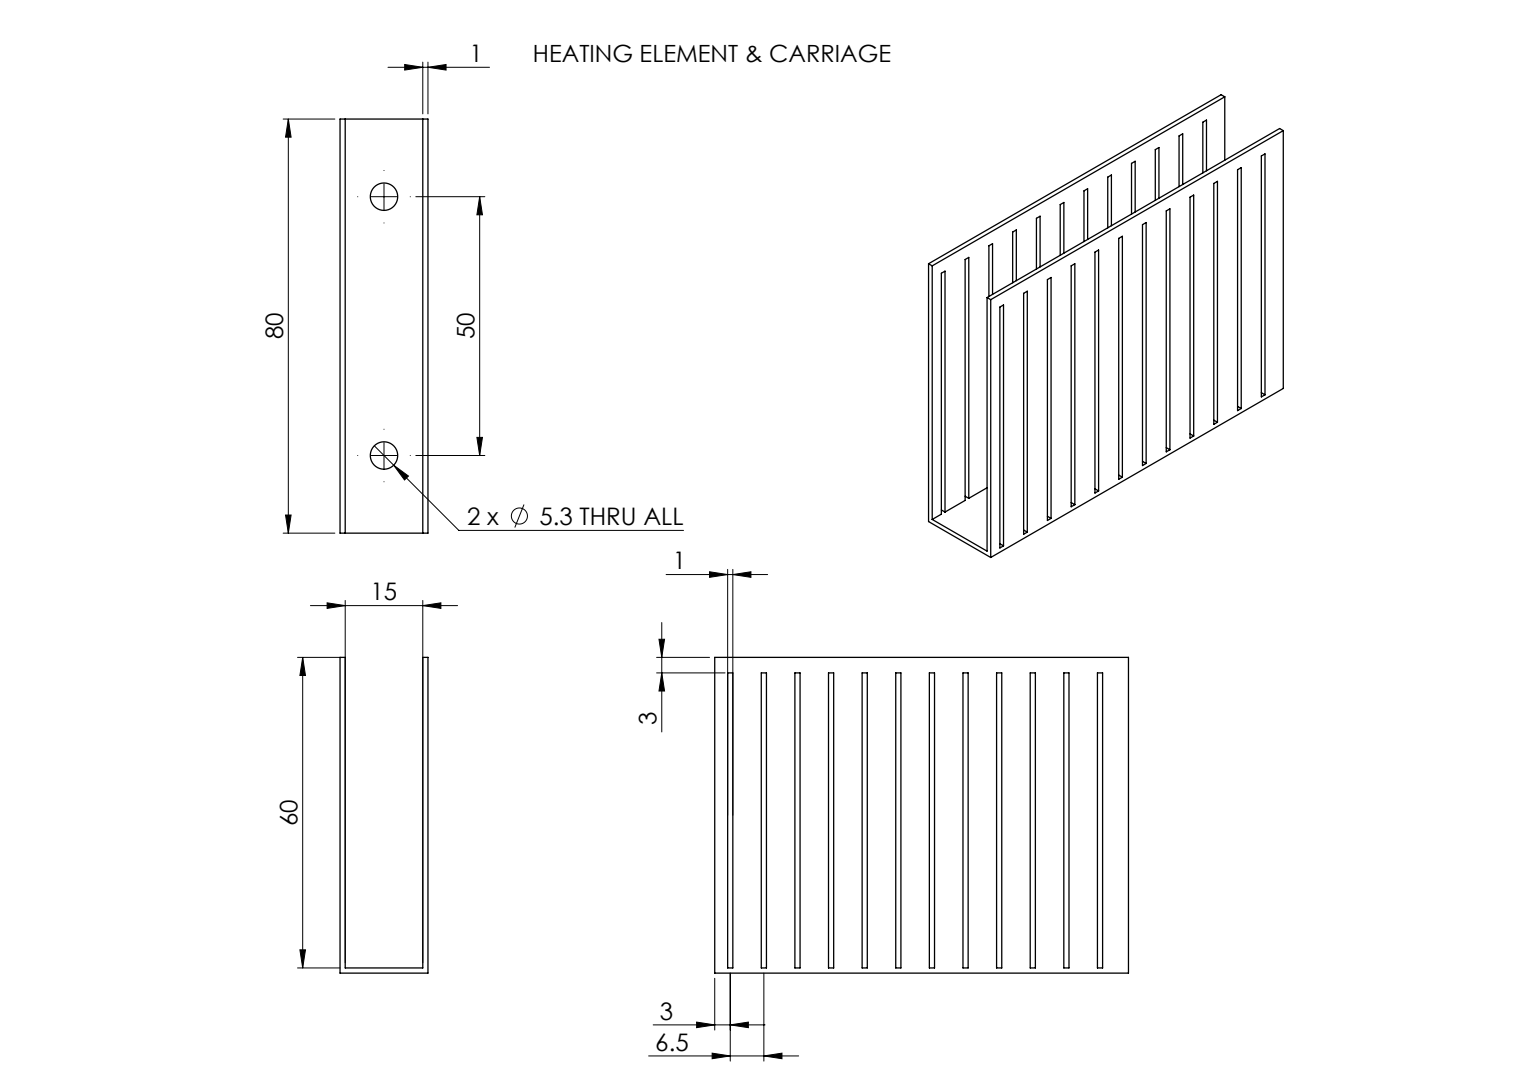
ISO-10303-21;
HEADER;
FILE_DESCRIPTION (('STEP AP214'),
    '1' );
FILE_NAME ('Heating Element & carriage.step',
    '2026-10-08T14:41:38',
    ( '' ),
    ( '' ),
    'SwSTEP 2.0',
    'SolidWorks 2026',
    '' );
FILE_SCHEMA (( 'AUTOMOTIVE_DESIGN' ));
ENDSEC;

DATA;
#2=VECTOR ( 'NONE', #8948, 1000.000000000000000 ) ;
#3=LINE ( 'NONE', #19320, #5933 ) ;
#8=DIRECTION ( 'NONE',  ( 0.000000000000000000, 0.000000000000000000, -1.000000000000000000 ) ) ;
#9=VERTEX_POINT ( 'NONE', #9196 ) ;
#11=VERTEX_POINT ( 'NONE', #7634 ) ;
#14=LINE ( 'NONE', #16487, #359 ) ;
#15=PRODUCT_CONTEXT ( 'NONE', #3327, 'mechanical' ) ;
#16=CARTESIAN_POINT ( 'NONE',  ( -25.00000000000000000, 53.00000000000000711, 30.00000000000000000 ) ) ;
#17=EDGE_CURVE ( 'NONE', #5613, #1380, #13300, .T. ) ;
#19=AXIS2_PLACEMENT_3D ( 'NONE', #7359, #17758, #4328 ) ;
#24=ORIENTED_EDGE ( 'NONE', *, *, #7353, .F. ) ;
#35=DIRECTION ( 'NONE',  ( -1.000000000000000000, 0.000000000000000000, -0.000000000000000000 ) ) ;
#39=CARTESIAN_POINT ( 'NONE',  ( -25.00000000000000000, 53.00000000000000711, -11.49999999999999645 ) ) ;
#46=PLANE ( 'NONE',  #8954 ) ;
#47=AXIS2_PLACEMENT_3D ( 'NONE', #8306, #16043, #2603 ) ;
#49=EDGE_LOOP ( 'NONE', ( #2329, #11638, #12440, #4824 ) ) ;
#60=CARTESIAN_POINT ( 'NONE',  ( -41.00000000000000711, 110.0000000000000000, 6.999999999999999112 ) ) ;
#64=EDGE_CURVE ( 'NONE', #9274, #14710, #15088, .T. ) ;
#67=AXIS2_PLACEMENT_3D ( 'NONE', #5864, #11526, #16244 ) ;
#76=VERTEX_POINT ( 'NONE', #16452 ) ;
#114=CARTESIAN_POINT ( 'NONE',  ( -24.00000000000000000, 53.00000000000000711, -18.00000000000000355 ) ) ;
#115=DIRECTION ( 'NONE',  ( 0.000000000000000000, 0.000000000000000000, -1.000000000000000000 ) ) ;
#130=ORIENTED_EDGE ( 'NONE', *, *, #2687, .F. ) ;
#132=EDGE_CURVE ( 'NONE', #16262, #13646, #5091, .T. ) ;
#141=DIRECTION ( 'NONE',  ( 0.000000000000000000, -1.000000000000000000, -0.000000000000000000 ) ) ;
#150=DIRECTION ( 'NONE',  ( 0.000000000000000000, 0.000000000000000000, 1.000000000000000000 ) ) ;
#173=ORIENTED_EDGE ( 'NONE', *, *, #18111, .T. ) ;
#176=CARTESIAN_POINT ( 'NONE',  ( -41.00000000000000711, 53.00000000000000711, 8.000000000000000000 ) ) ;
#184=VERTEX_POINT ( 'NONE', #3603 ) ;
#185=VERTEX_POINT ( 'NONE', #9574 ) ;
#193=VECTOR ( 'NONE', #5352, 1000.000000000000000 ) ;
#209=VERTEX_POINT ( 'NONE', #3697 ) ;
#218=CARTESIAN_POINT ( 'NONE',  ( -40.00000000000000000, 53.00000000000000711, 20.00000000000000000 ) ) ;
#221=LINE ( 'NONE', #319, #18355 ) ;
#230=EDGE_LOOP ( 'NONE', ( #8619, #14141, #10740, #17845 ) ) ;
#234=CARTESIAN_POINT ( 'NONE',  ( -40.00000000000000000, 53.00000000000000711, -32.00000000000000000 ) ) ;
#236=CARTESIAN_POINT ( 'NONE',  ( -41.00000000000000711, 53.00000000000000711, -45.00000000000000000 ) ) ;
#249=LINE ( 'NONE', #3293, #1715 ) ;
#254=CARTESIAN_POINT ( 'NONE',  ( -41.00000000000000711, 53.00000000000000711, 13.50000000000000000 ) ) ;
#258=EDGE_CURVE ( 'NONE', #10251, #6518, #1845, .T. ) ;
#277=ORIENTED_EDGE ( 'NONE', *, *, #8740, .F. ) ;
#279=CARTESIAN_POINT ( 'NONE',  ( -24.00000000000000711, 53.00000000000000711, -18.00000000000000000 ) ) ;
#280=EDGE_CURVE ( 'NONE', #3613, #17642, #1950, .T. ) ;
#285=EDGE_LOOP ( 'NONE', ( #7432, #10877, #13688, #10122 ) ) ;
#291=VERTEX_POINT ( 'NONE', #667 ) ;
#304=LINE ( 'NONE', #9218, #18172 ) ;
#309=LINE ( 'NONE', #12357, #13947 ) ;
#310=VECTOR ( 'NONE', #16083, 1000.000000000000000 ) ;
#313=VECTOR ( 'NONE', #8610, 1000.000000000000000 ) ;
#319=CARTESIAN_POINT ( 'NONE',  ( -40.00000000000000711, 110.0000000000000000, 30.00000000000000000 ) ) ;
#332=CARTESIAN_POINT ( 'NONE',  ( -25.00000000000000000, 113.0000000000000000, 30.00000000000000000 ) ) ;
#338=VECTOR ( 'NONE', #15976, 1000.000000000000000 ) ;
#342=AXIS2_PLACEMENT_3D ( 'NONE', #8168, #7978, #714 ) ;
#343=EDGE_LOOP ( 'NONE', ( #9305, #13118, #10006, #16658 ) ) ;
#349=FACE_OUTER_BOUND ( 'NONE', #18147, .T. ) ;
#353=DIRECTION ( 'NONE',  ( 1.000000000000000000, -0.000000000000000000, -0.000000000000000000 ) ) ;
#358=DIRECTION ( 'NONE',  ( 1.000000000000000000, -0.000000000000000000, -0.000000000000000000 ) ) ;
#359=VECTOR ( 'NONE', #18061, 1000.000000000000000 ) ;
#361=CARTESIAN_POINT ( 'NONE',  ( -41.00000000000000711, 53.00000000000000711, 27.50000000000000000 ) ) ;
#364=ORIENTED_EDGE ( 'NONE', *, *, #7937, .T. ) ;
#368=ORIENTED_EDGE ( 'NONE', *, *, #14861, .F. ) ;
#379=CARTESIAN_POINT ( 'NONE',  ( -25.00000000000000000, 53.00000000000000711, 30.00000000000000000 ) ) ;
#381=ORIENTED_EDGE ( 'NONE', *, *, #2414, .F. ) ;
#409=DIRECTION ( 'NONE',  ( 1.000000000000000000, -0.000000000000000000, -0.000000000000000000 ) ) ;
#412=CARTESIAN_POINT ( 'NONE',  ( -41.00000000000000711, 53.00000000000000711, 6.999999999999999112 ) ) ;
#417=DIRECTION ( 'NONE',  ( -0.000000000000000000, 1.000000000000000000, -0.000000000000000000 ) ) ;
#430=CARTESIAN_POINT ( 'NONE',  ( -41.00000000000000711, 110.0000000000000000, -6.000000000000001776 ) ) ;
#432=DIRECTION ( 'NONE',  ( 1.000000000000000000, -0.000000000000000000, -0.000000000000000000 ) ) ;
#436=EDGE_CURVE ( 'NONE', #19394, #6733, #8675, .T. ) ;
#437=CARTESIAN_POINT ( 'NONE',  ( -41.00000000000000711, 110.0000000000000000, 20.00000000000000000 ) ) ;
#453=ADVANCED_FACE ( 'NONE', ( #1229 ), #11327, .T. ) ;
#464=DIRECTION ( 'NONE',  ( 0.000000000000000000, -1.000000000000000000, 0.000000000000000000 ) ) ;
#472=VECTOR ( 'NONE', #8947, 1000.000000000000000 ) ;
#474=DIRECTION ( 'NONE',  ( 0.000000000000000000, 0.000000000000000000, 1.000000000000000000 ) ) ;
#478=LINE ( 'NONE', #15666, #7219 ) ;
#480=ORIENTED_EDGE ( 'NONE', *, *, #9077, .T. ) ;
#485=ORIENTED_EDGE ( 'NONE', *, *, #2062, .T. ) ;
#487=ORIENTED_EDGE ( 'NONE', *, *, #6763, .T. ) ;
#494=ORIENTED_EDGE ( 'NONE', *, *, #810, .F. ) ;
#499=CARTESIAN_POINT ( 'NONE',  ( -25.00000000000000711, 53.00000000000000711, 1.500000000000001332 ) ) ;
#501=FACE_BOUND ( 'NONE', #14667, .T. ) ;
#506=CARTESIAN_POINT ( 'NONE',  ( -41.00000000000000711, 53.00000000000000711, -45.00000000000000000 ) ) ;
#509=ORIENTED_EDGE ( 'NONE', *, *, #2274, .F. ) ;
#512=CARTESIAN_POINT ( 'NONE',  ( -41.00000000000000711, 53.00000000000000711, 26.50000000000000000 ) ) ;
#520=ORIENTED_EDGE ( 'NONE', *, *, #14321, .T. ) ;
#522=ORIENTED_EDGE ( 'NONE', *, *, #3988, .F. ) ;
#523=DIRECTION ( 'NONE',  ( -1.156482317317871478E-16, 1.000000000000000000, 0.000000000000000000 ) ) ;
#525=LINE ( 'NONE', #11565, #11597 ) ;
#529=VECTOR ( 'NONE', #12275, 1000.000000000000000 ) ;
#530=VECTOR ( 'NONE', #4637, 1000.000000000000000 ) ;
#532=DIRECTION ( 'NONE',  ( 0.000000000000000000, 0.000000000000000000, -1.000000000000000000 ) ) ;
#534=DIRECTION ( 'NONE',  ( 1.000000000000000000, -0.000000000000000000, -0.000000000000000000 ) ) ;
#564=LINE ( 'NONE', #18228, #7201 ) ;
#588=CARTESIAN_POINT ( 'NONE',  ( -41.00000000000000711, 53.00000000000000711, -24.49999999999999645 ) ) ;
#592=DIRECTION ( 'NONE',  ( -1.156482317317871478E-16, 1.000000000000000000, 0.000000000000000000 ) ) ;
#593=FACE_BOUND ( 'NONE', #7659, .T. ) ;
#599=VECTOR ( 'NONE', #2972, 1000.000000000000000 ) ;
#601=DIRECTION ( 'NONE',  ( 0.000000000000000000, 0.000000000000000000, -1.000000000000000000 ) ) ;
#605=ORIENTED_EDGE ( 'NONE', *, *, #6639, .T. ) ;
#612=VECTOR ( 'NONE', #474, 1000.000000000000000 ) ;
#617=ADVANCED_FACE ( 'NONE', ( #14763 ), #16425, .T. ) ;
#621=VECTOR ( 'NONE', #523, 1000.000000000000000 ) ;
#622=LINE ( 'NONE', #15618, #18616 ) ;
#625=EDGE_CURVE ( 'NONE', #3704, #982, #6141, .T. ) ;
#626=VECTOR ( 'NONE', #2257, 1000.000000000000000 ) ;
#630=AXIS2_PLACEMENT_3D ( 'NONE', #16972, #17154, #15490 ) ;
#634=VECTOR ( 'NONE', #11787, 1000.000000000000000 ) ;
#635=LINE ( 'NONE', #15629, #18156 ) ;
#643=CARTESIAN_POINT ( 'NONE',  ( -24.00000000000000000, 113.0000000000000000, 30.00000000000000000 ) ) ;
#645=VECTOR ( 'NONE', #16601, 1000.000000000000000 ) ;
#649=VECTOR ( 'NONE', #15920, 1000.000000000000000 ) ;
#650=ORIENTED_EDGE ( 'NONE', *, *, #9548, .F. ) ;
#656=EDGE_CURVE ( 'NONE', #10380, #10947, #3089, .T. ) ;
#658=FACE_OUTER_BOUND ( 'NONE', #6966, .T. ) ;
#659=EDGE_CURVE ( 'NONE', #16948, #10794, #10433, .T. ) ;
#664=EDGE_LOOP ( 'NONE', ( #7813, #9877, #10932, #13103 ) ) ;
#667=CARTESIAN_POINT ( 'NONE',  ( -41.00000000000000711, 110.0000000000000000, -32.00000000000000000 ) ) ;
#668=VECTOR ( 'NONE', #17005, 1000.000000000000000 ) ;
#670=CARTESIAN_POINT ( 'NONE',  ( -25.00000000000000000, 110.0000000000000000, 30.00000000000000000 ) ) ;
#678=ORIENTED_EDGE ( 'NONE', *, *, #14772, .F. ) ;
#681=ORIENTED_EDGE ( 'NONE', *, *, #18605, .T. ) ;
#689=ORIENTED_EDGE ( 'NONE', *, *, #866, .F. ) ;
#691=DIRECTION ( 'NONE',  ( 0.000000000000000000, -1.000000000000000000, -0.000000000000000000 ) ) ;
#692=ORIENTED_EDGE ( 'NONE', *, *, #7602, .T. ) ;
#695=CARTESIAN_POINT ( 'NONE',  ( -41.00000000000000711, 110.0000000000000000, -5.000000000000000888 ) ) ;
#707=ORIENTED_EDGE ( 'NONE', *, *, #2186, .T. ) ;
#710=ORIENTED_EDGE ( 'NONE', *, *, #11906, .T. ) ;
#714=DIRECTION ( 'NONE',  ( -1.000000000000000000, 0.000000000000000000, -0.000000000000000000 ) ) ;
#722=LINE ( 'NONE', #6702, #12252 ) ;
#726=ORIENTED_EDGE ( 'NONE', *, *, #2307, .T. ) ;
#733=CARTESIAN_POINT ( 'NONE',  ( -40.00000000000000000, 53.00000000000000711, 13.50000000000000000 ) ) ;
#735=DIRECTION ( 'NONE',  ( 0.000000000000000000, 0.000000000000000000, -1.000000000000000000 ) ) ;
#738=CARTESIAN_POINT ( 'NONE',  ( -41.00000000000000711, 53.00000000000000711, -19.00000000000000000 ) ) ;
#755=DIRECTION ( 'NONE',  ( 0.000000000000000000, 0.000000000000000000, -1.000000000000000000 ) ) ;
#758=VECTOR ( 'NONE', #9249, 1000.000000000000000 ) ;
#759=DIRECTION ( 'NONE',  ( 1.000000000000000000, -0.000000000000000000, -0.000000000000000000 ) ) ;
#760=EDGE_CURVE ( 'NONE', #2931, #1646, #7705, .T. ) ;
#766=ORIENTED_EDGE ( 'NONE', *, *, #2307, .F. ) ;
#767=ORIENTED_EDGE ( 'NONE', *, *, #16915, .F. ) ;
#773=LINE ( 'NONE', #2428, #11566 ) ;
#776=DIRECTION ( 'NONE',  ( 1.000000000000000000, -0.000000000000000000, -0.000000000000000000 ) ) ;
#778=DIRECTION ( 'NONE',  ( 0.000000000000000000, -1.000000000000000000, 0.000000000000000000 ) ) ;
#783=CARTESIAN_POINT ( 'NONE',  ( -40.00000000000000711, 113.0000000000000000, 6.999999999999999112 ) ) ;
#790=AXIS2_PLACEMENT_3D ( 'NONE', #8176, #5235, #14146 ) ;
#798=LINE ( 'NONE', #18747, #17206 ) ;
#802=VECTOR ( 'NONE', #3506, 1000.000000000000000 ) ;
#803=CARTESIAN_POINT ( 'NONE',  ( -41.00000000000000711, 110.0000000000000000, -5.000000000000000888 ) ) ;
#804=ORIENTED_EDGE ( 'NONE', *, *, #13435, .F. ) ;
#809=CARTESIAN_POINT ( 'NONE',  ( -41.00000000000000711, 113.0000000000000000, 30.00000000000000000 ) ) ;
#810=EDGE_CURVE ( 'NONE', #15519, #4628, #9647, .T. ) ;
#824=VECTOR ( 'NONE', #2637, 1000.000000000000000 ) ;
#836=VECTOR ( 'NONE', #15353, 1000.000000000000000 ) ;
#853=VERTEX_POINT ( 'NONE', #2582 ) ;
#857=ORIENTED_EDGE ( 'NONE', *, *, #3921, .T. ) ;
#864=CARTESIAN_POINT ( 'NONE',  ( -41.00000000000000711, 110.0000000000000000, 21.00000000000000000 ) ) ;
#866=EDGE_CURVE ( 'NONE', #19283, #17238, #6714, .T. ) ;
#868=PLANE ( 'NONE',  #16631 ) ;
#870=FACE_OUTER_BOUND ( 'NONE', #10505, .T. ) ;
#876=EDGE_CURVE ( 'NONE', #15646, #8090, #3962, .T. ) ;
#880=ORIENTED_EDGE ( 'NONE', *, *, #12234, .F. ) ;
#883=VECTOR ( 'NONE', #3984, 1000.000000000000000 ) ;
#890=EDGE_LOOP ( 'NONE', ( #5514, #15277, #16400, #16858 ) ) ;
#897=ADVANCED_FACE ( 'NONE', ( #8562 ), #18770, .T. ) ;
#901=SURFACE_STYLE_USAGE ( .BOTH. , #5326 ) ;
#906=EDGE_LOOP ( 'NONE', ( #5274, #17895, #7595, #10353 ) ) ;
#913=LINE ( 'NONE', #17382, #14105 ) ;
#916=LINE ( 'NONE', #1204, #4548 ) ;
#927=CARTESIAN_POINT ( 'NONE',  ( -41.00000000000000711, 110.0000000000000000, 14.50000000000000000 ) ) ;
#928=VECTOR ( 'NONE', #4321, 1000.000000000000000 ) ;
#934=PLANE ( 'NONE',  #16670 ) ;
#940=DIRECTION ( 'NONE',  ( 1.000000000000000000, 1.156482317317871478E-16, -0.000000000000000000 ) ) ;
#941=VECTOR ( 'NONE', #1797, 1000.000000000000000 ) ;
#943=LINE ( 'NONE', #17412, #883 ) ;
#944=FACE_OUTER_BOUND ( 'NONE', #1471, .T. ) ;
#950=ORIENTED_EDGE ( 'NONE', *, *, #18620, .F. ) ;
#952=FILL_AREA_STYLE_COLOUR ( '', #15246 ) ;
#967=AXIS2_PLACEMENT_3D ( 'NONE', #13487, #8976, #17705 ) ;
#968=FACE_OUTER_BOUND ( 'NONE', #890, .T. ) ;
#977=VECTOR ( 'NONE', #19393, 1000.000000000000000 ) ;
#978=CARTESIAN_POINT ( 'NONE',  ( -24.00000000000000711, 53.00000000000000711, 14.50000000000000000 ) ) ;
#981=EDGE_LOOP ( 'NONE', ( #1286, #11849, #18751, #17689 ) ) ;
#982=VERTEX_POINT ( 'NONE', #15919 ) ;
#993=VERTEX_POINT ( 'NONE', #12965 ) ;
#995=DIRECTION ( 'NONE',  ( -0.000000000000000000, -0.000000000000000000, -1.000000000000000000 ) ) ;
#998=DIRECTION ( 'NONE',  ( -1.156482317317871478E-16, 1.000000000000000000, 0.000000000000000000 ) ) ;
#1006=ADVANCED_FACE ( 'NONE', ( #4256 ), #4553, .F. ) ;
#1009=ORIENTED_EDGE ( 'NONE', *, *, #16981, .F. ) ;
#1017=DIRECTION ( 'NONE',  ( -0.000000000000000000, -0.000000000000000000, -1.000000000000000000 ) ) ;
#1029=LINE ( 'NONE', #3587, #8038 ) ;
#1034=PLANE ( 'NONE',  #12270 ) ;
#1042=LINE ( 'NONE', #15761, #17575 ) ;
#1049=VERTEX_POINT ( 'NONE', #13256 ) ;
#1050=VERTEX_POINT ( 'NONE', #3071 ) ;
#1054=CARTESIAN_POINT ( 'NONE',  ( -24.00000000000000000, 110.0000000000000000, 30.00000000000000000 ) ) ;
#1057=VERTEX_POINT ( 'NONE', #14943 ) ;
#1058=DIRECTION ( 'NONE',  ( 1.000000000000000000, -0.000000000000000000, -0.000000000000000000 ) ) ;
#1059=EDGE_LOOP ( 'NONE', ( #16999, #10652, #8275, #15172 ) ) ;
#1075=DIRECTION ( 'NONE',  ( 0.000000000000000000, 0.000000000000000000, 1.000000000000000000 ) ) ;
#1077=AXIS2_PLACEMENT_3D ( 'NONE', #3070, #4653, #6219 ) ;
#1094=CARTESIAN_POINT ( 'NONE',  ( -41.00000000000000711, 53.00000000000000711, 0.5000000000000004441 ) ) ;
#1096=PLANE ( 'NONE',  #13026 ) ;
#1106=EDGE_CURVE ( 'NONE', #3347, #18273, #16111, .T. ) ;
#1112=DIRECTION ( 'NONE',  ( -1.000000000000000000, 0.000000000000000000, -0.000000000000000000 ) ) ;
#1117=VECTOR ( 'NONE', #5853, 1000.000000000000000 ) ;
#1135=EDGE_CURVE ( 'NONE', #5597, #2911, #5918, .T. ) ;
#1141=VECTOR ( 'NONE', #9980, 1000.000000000000000 ) ;
#1143=DIRECTION ( 'NONE',  ( 1.000000000000000000, -0.000000000000000000, -0.000000000000000000 ) ) ;
#1161=LINE ( 'NONE', #15875, #6006 ) ;
#1167=DIRECTION ( 'NONE',  ( -0.000000000000000000, -0.000000000000000000, -1.000000000000000000 ) ) ;
#1173=ORIENTED_EDGE ( 'NONE', *, *, #3972, .F. ) ;
#1180=LINE ( 'NONE', #3749, #310 ) ;
#1184=CARTESIAN_POINT ( 'NONE',  ( -25.00000000000000000, 53.00000000000000711, -6.000000000000005329 ) ) ;
#1196=ADVANCED_FACE ( 'NONE', ( #5210 ), #3442, .T. ) ;
#1200=VERTEX_POINT ( 'NONE', #15692 ) ;
#1204=CARTESIAN_POINT ( 'NONE',  ( -24.00000000000000000, 53.00000000000000711, 30.00000000000000000 ) ) ;
#1212=DIRECTION ( 'NONE',  ( -1.156482317317871478E-16, 1.000000000000000000, 0.000000000000000000 ) ) ;
#1214=PLANE ( 'NONE',  #18980 ) ;
#1215=VECTOR ( 'NONE', #16726, 1000.000000000000000 ) ;
#1228=VECTOR ( 'NONE', #16896, 1000.000000000000000 ) ;
#1229=FACE_OUTER_BOUND ( 'NONE', #13960, .T. ) ;
#1233=DIRECTION ( 'NONE',  ( -1.000000000000000000, 0.000000000000000000, -0.000000000000000000 ) ) ;
#1236=VECTOR ( 'NONE', #8624, 1000.000000000000000 ) ;
#1241=EDGE_LOOP ( 'NONE', ( #11948, #10912, #17945, #1283, #1566, #9146, #520, #3733, #14803, #5855, #6245, #19227, #15301, #8219, #16469, #17525, #16503, #381, #18039, #7623, #19032, #7521, #5716, #16047, #880, #13494, #16643, #2727, #18760, #1009, #4004, #5780, #2228, #3499, #10444, #726, #9450, #8717, #10174, #15705, #13406, #9481, #5037, #3504, #6291, #11719, #4592, #1657, #18703, #12860, #1476, #9601, #14968, #5586, #12915, #1586, #15890, #10759, #2179, #173, #10361, #17542, #16573, #15103, #6064, #17514, #2445, #2873, #16154, #689, #364, #9395, #4625, #24, #10077, #11238, #16268, #11151, #19225, #9913, #15765, #10497, #6485, #19212, #5003, #15390, #7620, #10672, #10260, #6196, #7749, #1376, #485, #13117, #18781, #6011, #17055, #9084, #1773, #1677 ) ) ;
#1247=EDGE_LOOP ( 'NONE', ( #7632, #14235, #9399, #2813 ) ) ;
#1250=EDGE_CURVE ( 'NONE', #19005, #3857, #12736, .T. ) ;
#1253=AXIS2_PLACEMENT_3D ( 'NONE', #15002, #13527, #2941 ) ;
#1258=LINE ( 'NONE', #11829, #15370 ) ;
#1260=AXIS2_PLACEMENT_3D ( 'NONE', #5822, #17678, #1112 ) ;
#1273=VERTEX_POINT ( 'NONE', #15410 ) ;
#1274=EDGE_LOOP ( 'NONE', ( #8686, #17929, #678, #19092 ) ) ;
#1276=DIRECTION ( 'NONE',  ( 0.000000000000000000, 0.000000000000000000, -1.000000000000000000 ) ) ;
#1278=ORIENTED_EDGE ( 'NONE', *, *, #6601, .F. ) ;
#1281=VECTOR ( 'NONE', #16758, 1000.000000000000000 ) ;
#1282=CARTESIAN_POINT ( 'NONE',  ( -25.00000000000000000, 53.00000000000000711, 30.00000000000000000 ) ) ;
#1283=ORIENTED_EDGE ( 'NONE', *, *, #9412, .T. ) ;
#1286=ORIENTED_EDGE ( 'NONE', *, *, #9886, .T. ) ;
#1290=ORIENTED_EDGE ( 'NONE', *, *, #14321, .F. ) ;
#1291=CARTESIAN_POINT ( 'NONE',  ( -24.00000000000000711, 53.00000000000000711, 21.00000000000000000 ) ) ;
#1295=EDGE_CURVE ( 'NONE', #12537, #17031, #12824, .T. ) ;
#1310=VECTOR ( 'NONE', #18785, 1000.000000000000000 ) ;
#1312=ORIENTED_EDGE ( 'NONE', *, *, #15617, .F. ) ;
#1314=ORIENTED_EDGE ( 'NONE', *, *, #13054, .F. ) ;
#1317=DIRECTION ( 'NONE',  ( 0.000000000000000000, 0.000000000000000000, 1.000000000000000000 ) ) ;
#1335=DIRECTION ( 'NONE',  ( 0.000000000000000000, 0.000000000000000000, -1.000000000000000000 ) ) ;
#1337=DIRECTION ( 'NONE',  ( 1.000000000000000000, -0.000000000000000000, -0.000000000000000000 ) ) ;
#1342=ADVANCED_FACE ( 'NONE', ( #6586, #5295, #5122 ), #14307, .F. ) ;
#1343=CARTESIAN_POINT ( 'NONE',  ( -40.00000000000000711, 110.0000000000000000, 8.000000000000000000 ) ) ;
#1350=VERTEX_POINT ( 'NONE', #499 ) ;
#1352=CARTESIAN_POINT ( 'NONE',  ( -24.00000000000000000, 53.00000000000000711, 30.00000000000000000 ) ) ;
#1356=ORIENTED_EDGE ( 'NONE', *, *, #9299, .F. ) ;
#1368=CARTESIAN_POINT ( 'NONE',  ( -41.00000000000000711, 53.00000000000000711, 21.00000000000000000 ) ) ;
#1369=LINE ( 'NONE', #11947, #8007 ) ;
#1370=VERTEX_POINT ( 'NONE', #10978 ) ;
#1376=ORIENTED_EDGE ( 'NONE', *, *, #4289, .T. ) ;
#1380=VERTEX_POINT ( 'NONE', #9607 ) ;
#1384=EDGE_CURVE ( 'NONE', #7148, #3017, #15594, .T. ) ;
#1385=CARTESIAN_POINT ( 'NONE',  ( -25.00000000000000000, 113.0000000000000000, 30.00000000000000000 ) ) ;
#1386=ORIENTED_EDGE ( 'NONE', *, *, #13706, .F. ) ;
#1389=LINE ( 'NONE', #1492, #17894 ) ;
#1392=LINE ( 'NONE', #12066, #10527 ) ;
#1400=EDGE_CURVE ( 'NONE', #5597, #13388, #7241, .T. ) ;
#1408=FACE_OUTER_BOUND ( 'NONE', #2091, .T. ) ;
#1418=CARTESIAN_POINT ( 'NONE',  ( -25.00000000000000000, 53.00000000000000711, 1.500000000000001332 ) ) ;
#1421=ORIENTED_EDGE ( 'NONE', *, *, #15282, .F. ) ;
#1423=EDGE_CURVE ( 'NONE', #12114, #17652, #17346, .T. ) ;
#1425=DIRECTION ( 'NONE',  ( 0.000000000000000000, 0.000000000000000000, -1.000000000000000000 ) ) ;
#1439=FACE_OUTER_BOUND ( 'NONE', #11726, .T. ) ;
#1445=VECTOR ( 'NONE', #9654, 1000.000000000000000 ) ;
#1465=AXIS2_PLACEMENT_3D ( 'NONE', #512, #7971, #1987 ) ;
#1467=AXIS2_PLACEMENT_3D ( 'NONE', #4932, #18736, #5216 ) ;
#1468=LINE ( 'NONE', #18234, #16955 ) ;
#1471=EDGE_LOOP ( 'NONE', ( #15796, #4172, #5621, #13747 ) ) ;
#1475=CARTESIAN_POINT ( 'NONE',  ( -41.00000000000000711, 53.00000000000000711, -24.49999999999999645 ) ) ;
#1476=ORIENTED_EDGE ( 'NONE', *, *, #15747, .T. ) ;
#1479=EDGE_CURVE ( 'NONE', #4790, #1553, #4307, .T. ) ;
#1485=CARTESIAN_POINT ( 'NONE',  ( -24.00000000000000000, 52.00000000000000711, 30.00000000000000000 ) ) ;
#1492=CARTESIAN_POINT ( 'NONE',  ( -24.00000000000000000, 110.0000000000000000, 30.00000000000000000 ) ) ;
#1510=ORIENTED_EDGE ( 'NONE', *, *, #3396, .T. ) ;
#1518=EDGE_CURVE ( 'NONE', #3704, #12114, #13114, .T. ) ;
#1520=FACE_OUTER_BOUND ( 'NONE', #6704, .T. ) ;
#1532=DIRECTION ( 'NONE',  ( 1.000000000000000000, -0.000000000000000000, -0.000000000000000000 ) ) ;
#1534=CARTESIAN_POINT ( 'NONE',  ( -41.00000000000000711, 53.00000000000000711, 8.000000000000000000 ) ) ;
#1547=ORIENTED_EDGE ( 'NONE', *, *, #16219, .T. ) ;
#1553=VERTEX_POINT ( 'NONE', #5578 ) ;
#1566=ORIENTED_EDGE ( 'NONE', *, *, #11894, .F. ) ;
#1572=VERTEX_POINT ( 'NONE', #2625 ) ;
#1574=ORIENTED_EDGE ( 'NONE', *, *, #15403, .F. ) ;
#1577=AXIS2_PLACEMENT_3D ( 'NONE', #5121, #15303, #6392 ) ;
#1580=ORIENTED_EDGE ( 'NONE', *, *, #12249, .T. ) ;
#1582=EDGE_CURVE ( 'NONE', #16384, #14586, #19204, .T. ) ;
#1586=ORIENTED_EDGE ( 'NONE', *, *, #13525, .T. ) ;
#1589=LINE ( 'NONE', #114, #9423 ) ;
#1603=VECTOR ( 'NONE', #13229, 1000.000000000000000 ) ;
#1608=VECTOR ( 'NONE', #13834, 1000.000000000000000 ) ;
#1616=ADVANCED_FACE ( 'NONE', ( #10368 ), #17935, .T. ) ;
#1619=EDGE_CURVE ( 'NONE', #15030, #5693, #13303, .T. ) ;
#1620=AXIS2_PLACEMENT_3D ( 'NONE', #4076, #940, #8302 ) ;
#1623=AXIS2_PLACEMENT_3D ( 'NONE', #18592, #13139, #4034 ) ;
#1631=CARTESIAN_POINT ( 'NONE',  ( -24.00000000000000000, 53.00000000000000711, 30.00000000000000000 ) ) ;
#1634=EDGE_CURVE ( 'NONE', #19128, #291, #16456, .T. ) ;
#1639=LINE ( 'NONE', #12205, #13397 ) ;
#1646=VERTEX_POINT ( 'NONE', #279 ) ;
#1651=ORIENTED_EDGE ( 'NONE', *, *, #13062, .T. ) ;
#1653=LINE ( 'NONE', #1352, #15830 ) ;
#1657=ORIENTED_EDGE ( 'NONE', *, *, #14988, .T. ) ;
#1659=ORIENTED_EDGE ( 'NONE', *, *, #17, .T. ) ;
#1661=VERTEX_POINT ( 'NONE', #2925 ) ;
#1662=VERTEX_POINT ( 'NONE', #12233 ) ;
#1666=DIRECTION ( 'NONE',  ( 0.000000000000000000, 0.000000000000000000, -1.000000000000000000 ) ) ;
#1673=VERTEX_POINT ( 'NONE', #10756 ) ;
#1677=ORIENTED_EDGE ( 'NONE', *, *, #16225, .F. ) ;
#1685=CARTESIAN_POINT ( 'NONE',  ( -25.00000000000000000, 110.0000000000000000, 30.00000000000000000 ) ) ;
#1696=CARTESIAN_POINT ( 'NONE',  ( -41.00000000000000711, 53.00000000000000711, -32.00000000000000000 ) ) ;
#1705=VECTOR ( 'NONE', #14150, 1000.000000000000000 ) ;
#1715=VECTOR ( 'NONE', #6233, 1000.000000000000000 ) ;
#1725=DIRECTION ( 'NONE',  ( 0.000000000000000000, -1.000000000000000000, 0.000000000000000000 ) ) ;
#1727=DIRECTION ( 'NONE',  ( 0.000000000000000000, 0.000000000000000000, 1.000000000000000000 ) ) ;
#1728=EDGE_LOOP ( 'NONE', ( #18520, #15861, #6751, #2742 ) ) ;
#1734=DIRECTION ( 'NONE',  ( 1.000000000000000000, -0.000000000000000000, -0.000000000000000000 ) ) ;
#1735=ORIENTED_EDGE ( 'NONE', *, *, #7505, .F. ) ;
#1740=ORIENTED_EDGE ( 'NONE', *, *, #6968, .F. ) ;
#1751=DIRECTION ( 'NONE',  ( 0.000000000000000000, 0.000000000000000000, 1.000000000000000000 ) ) ;
#1752=DIRECTION ( 'NONE',  ( -0.000000000000000000, -0.000000000000000000, -1.000000000000000000 ) ) ;
#1756=CARTESIAN_POINT ( 'NONE',  ( -25.00000000000000000, 110.0000000000000000, 27.50000000000000000 ) ) ;
#1759=VECTOR ( 'NONE', #10320, 1000.000000000000000 ) ;
#1762=ORIENTED_EDGE ( 'NONE', *, *, #6968, .T. ) ;
#1767=VERTEX_POINT ( 'NONE', #9576 ) ;
#1768=ORIENTED_EDGE ( 'NONE', *, *, #5180, .F. ) ;
#1773=ORIENTED_EDGE ( 'NONE', *, *, #13926, .T. ) ;
#1780=ORIENTED_EDGE ( 'NONE', *, *, #14871, .T. ) ;
#1785=DIRECTION ( 'NONE',  ( 0.000000000000000000, -1.000000000000000000, -0.000000000000000000 ) ) ;
#1786=LINE ( 'NONE', #16, #13514 ) ;
#1791=AXIS2_PLACEMENT_3D ( 'NONE', #13713, #4815, #7646 ) ;
#1793=VERTEX_POINT ( 'NONE', #3414 ) ;
#1797=DIRECTION ( 'NONE',  ( 1.000000000000000000, -0.000000000000000000, -0.000000000000000000 ) ) ;
#1799=DIRECTION ( 'NONE',  ( 0.000000000000000000, 0.000000000000000000, -1.000000000000000000 ) ) ;
#1804=CARTESIAN_POINT ( 'NONE',  ( -41.00000000000000711, 53.00000000000000711, -6.000000000000001776 ) ) ;
#1805=CARTESIAN_POINT ( 'NONE',  ( -40.00000000000000000, 53.00000000000000711, 30.00000000000000000 ) ) ;
#1832=VERTEX_POINT ( 'NONE', #6368 ) ;
#1838=DIRECTION ( 'NONE',  ( 0.000000000000000000, 0.000000000000000000, -1.000000000000000000 ) ) ;
#1843=EDGE_LOOP ( 'NONE', ( #18532, #6957, #6275, #1278 ) ) ;
#1844=DIRECTION ( 'NONE',  ( 0.000000000000000000, 0.000000000000000000, -1.000000000000000000 ) ) ;
#1845=LINE ( 'NONE', #7831, #7893 ) ;
#1863=EDGE_LOOP ( 'NONE', ( #16180, #8342, #18695, #6665 ) ) ;
#1874=VERTEX_POINT ( 'NONE', #18525 ) ;
#1877=CARTESIAN_POINT ( 'NONE',  ( -40.00000000000000711, 53.00000000000000711, 8.000000000000000000 ) ) ;
#1878=EDGE_CURVE ( 'NONE', #1057, #15240, #18707, .T. ) ;
#1879=PLANE ( 'NONE',  #1577 ) ;
#1880=FACE_BOUND ( 'NONE', #1843, .T. ) ;
#1882=LINE ( 'NONE', #15501, #12863 ) ;
#1884=AXIS2_PLACEMENT_3D ( 'NONE', #13511, #17830, #3325 ) ;
#1890=ORIENTED_EDGE ( 'NONE', *, *, #760, .F. ) ;
#1893=ORIENTED_EDGE ( 'NONE', *, *, #12356, .T. ) ;
#1906=CARTESIAN_POINT ( 'NONE',  ( -41.00000000000000711, 53.00000000000000711, -44.00000000000000000 ) ) ;
#1908=AXIS2_PLACEMENT_3D ( 'NONE', #13111, #10073, #8704 ) ;
#1911=VECTOR ( 'NONE', #16871, 1000.000000000000000 ) ;
#1920=LINE ( 'NONE', #12489, #9763 ) ;
#1926=CARTESIAN_POINT ( 'NONE',  ( -25.00000000000000000, 53.00000000000000711, 30.00000000000000000 ) ) ;
#1929=DIRECTION ( 'NONE',  ( 0.000000000000000000, 0.000000000000000000, -1.000000000000000000 ) ) ;
#1931=AXIS2_PLACEMENT_3D ( 'NONE', #19330, #11859, #9026 ) ;
#1936=EDGE_LOOP ( 'NONE', ( #19049, #9020, #5575, #522 ) ) ;
#1939=ORIENTED_EDGE ( 'NONE', *, *, #18111, .F. ) ;
#1944=VECTOR ( 'NONE', #3202, 1000.000000000000000 ) ;
#1947=ORIENTED_EDGE ( 'NONE', *, *, #10082, .T. ) ;
#1950=LINE ( 'NONE', #8223, #12571 ) ;
#1958=EDGE_LOOP ( 'NONE', ( #17310, #17326, #17985, #14474 ) ) ;
#1987=DIRECTION ( 'NONE',  ( -1.000000000000000000, 0.000000000000000000, -0.000000000000000000 ) ) ;
#1992=FACE_OUTER_BOUND ( 'NONE', #7834, .T. ) ;
#1995=ORIENTED_EDGE ( 'NONE', *, *, #6514, .F. ) ;
#1996=LINE ( 'NONE', #7982, #621 ) ;
#2000=CARTESIAN_POINT ( 'NONE',  ( -41.00000000000000711, 53.00000000000000711, -45.00000000000000000 ) ) ;
#2008=( GEOMETRIC_REPRESENTATION_CONTEXT ( 3 ) GLOBAL_UNCERTAINTY_ASSIGNED_CONTEXT ( ( #3951 ) ) GLOBAL_UNIT_ASSIGNED_CONTEXT ( ( #4036, #14825, #15019 ) ) REPRESENTATION_CONTEXT ( 'NONE', 'WORKASPACE' ) );
#2009=CARTESIAN_POINT ( 'NONE',  ( -40.00000000000000000, 53.00000000000000711, -19.00000000000000000 ) ) ;
#2018=LINE ( 'NONE', #18305, #15413 ) ;
#2019=DIRECTION ( 'NONE',  ( -1.000000000000000000, 0.000000000000000000, -0.000000000000000000 ) ) ;
#2023=VECTOR ( 'NONE', #13859, 1000.000000000000000 ) ;
#2028=VERTEX_POINT ( 'NONE', #13078 ) ;
#2034=ORIENTED_EDGE ( 'NONE', *, *, #16815, .F. ) ;
#2038=DIRECTION ( 'NONE',  ( -1.156482317317871478E-16, 1.000000000000000000, 0.000000000000000000 ) ) ;
#2046=ORIENTED_EDGE ( 'NONE', *, *, #9532, .F. ) ;
#2049=CARTESIAN_POINT ( 'NONE',  ( -41.00000000000000711, 110.0000000000000000, 26.50000000000000000 ) ) ;
#2055=EDGE_CURVE ( 'NONE', #1767, #12537, #943, .T. ) ;
#2059=CARTESIAN_POINT ( 'NONE',  ( -24.00000000000000000, 110.0000000000000000, 19.99999999999999645 ) ) ;
#2062=EDGE_CURVE ( 'NONE', #17825, #12973, #3886, .T. ) ;
#2065=LINE ( 'NONE', #8056, #13773 ) ;
#2070=DIRECTION ( 'NONE',  ( 0.000000000000000000, 0.000000000000000000, -1.000000000000000000 ) ) ;
#2073=VECTOR ( 'NONE', #14569, 1000.000000000000000 ) ;
#2074=DIRECTION ( 'NONE',  ( 0.000000000000000000, 0.000000000000000000, -1.000000000000000000 ) ) ;
#2075=VECTOR ( 'NONE', #6244, 1000.000000000000000 ) ;
#2091=EDGE_LOOP ( 'NONE', ( #710, #277, #8234, #7127 ) ) ;
#2102=LINE ( 'NONE', #16904, #758 ) ;
#2106=ADVANCED_FACE ( 'NONE', ( #7115 ), #19078, .T. ) ;
#2112=DIRECTION ( 'NONE',  ( 0.000000000000000000, 0.000000000000000000, -1.000000000000000000 ) ) ;
#2120=CARTESIAN_POINT ( 'NONE',  ( -24.00000000000000000, 110.0000000000000000, 30.00000000000000000 ) ) ;
#2132=ORIENTED_EDGE ( 'NONE', *, *, #64, .T. ) ;
#2142=ORIENTED_EDGE ( 'NONE', *, *, #16219, .F. ) ;
#2146=VERTEX_POINT ( 'NONE', #17702 ) ;
#2150=VECTOR ( 'NONE', #11508, 1000.000000000000000 ) ;
#2153=CARTESIAN_POINT ( 'NONE',  ( -41.00000000000000711, 110.0000000000000000, -25.50000000000000000 ) ) ;
#2158=CARTESIAN_POINT ( 'NONE',  ( -41.00000000000000711, 53.00000000000000711, -6.000000000000001776 ) ) ;
#2162=CARTESIAN_POINT ( 'NONE',  ( -40.00000000000000000, 52.00000000000000711, 30.00000000000000000 ) ) ;
#2166=LINE ( 'NONE', #11258, #13473 ) ;
#2168=DIRECTION ( 'NONE',  ( 0.000000000000000000, 0.000000000000000000, 1.000000000000000000 ) ) ;
#2170=VERTEX_POINT ( 'NONE', #13675 ) ;
#2172=FACE_OUTER_BOUND ( 'NONE', #664, .T. ) ;
#2179=ORIENTED_EDGE ( 'NONE', *, *, #16558, .T. ) ;
#2181=CARTESIAN_POINT ( 'NONE',  ( -41.00000000000000711, 53.00000000000000711, 21.00000000000000000 ) ) ;
#2182=ORIENTED_EDGE ( 'NONE', *, *, #18397, .F. ) ;
#2184=FACE_OUTER_BOUND ( 'NONE', #3832, .T. ) ;
#2185=DIRECTION ( 'NONE',  ( 1.000000000000000000, -0.000000000000000000, -0.000000000000000000 ) ) ;
#2186=EDGE_CURVE ( 'NONE', #3115, #13282, #19372, .T. ) ;
#2203=EDGE_CURVE ( 'NONE', #1661, #2980, #5847, .T. ) ;
#2204=LINE ( 'NONE', #11019, #3903 ) ;
#2210=DIRECTION ( 'NONE',  ( 0.000000000000000000, -1.000000000000000000, 0.000000000000000000 ) ) ;
#2222=EDGE_CURVE ( 'NONE', #1572, #16704, #12004, .T. ) ;
#2228=ORIENTED_EDGE ( 'NONE', *, *, #12857, .F. ) ;
#2239=VERTEX_POINT ( 'NONE', #10630 ) ;
#2244=ORIENTED_EDGE ( 'NONE', *, *, #1518, .T. ) ;
#2245=ORIENTED_EDGE ( 'NONE', *, *, #8811, .F. ) ;
#2246=EDGE_CURVE ( 'NONE', #16262, #10297, #6239, .T. ) ;
#2252=DIRECTION ( 'NONE',  ( 0.000000000000000000, 0.000000000000000000, -1.000000000000000000 ) ) ;
#2257=DIRECTION ( 'NONE',  ( 0.000000000000000000, 0.000000000000000000, -1.000000000000000000 ) ) ;
#2266=VECTOR ( 'NONE', #15054, 1000.000000000000000 ) ;
#2269=VERTEX_POINT ( 'NONE', #2993 ) ;
#2274=EDGE_CURVE ( 'NONE', #9587, #17823, #1639, .T. ) ;
#2278=PLANE ( 'NONE',  #3150 ) ;
#2280=DIRECTION ( 'NONE',  ( -0.000000000000000000, -0.000000000000000000, -1.000000000000000000 ) ) ;
#2283=CARTESIAN_POINT ( 'NONE',  ( -40.00000000000000711, 113.0000000000000000, 1.500000000000001332 ) ) ;
#2285=FILL_AREA_STYLE ('',( #11474 ) ) ;
#2289=VERTEX_POINT ( 'NONE', #10435 ) ;
#2306=CARTESIAN_POINT ( 'NONE',  ( -41.00000000000000711, 110.0000000000000000, -12.50000000000000000 ) ) ;
#2307=EDGE_CURVE ( 'NONE', #14415, #6823, #17804, .T. ) ;
#2318=LINE ( 'NONE', #11505, #5595 ) ;
#2320=LINE ( 'NONE', #8304, #8422 ) ;
#2322=DIRECTION ( 'NONE',  ( -1.000000000000000000, 0.000000000000000000, -0.000000000000000000 ) ) ;
#2323=VECTOR ( 'NONE', #7393, 1000.000000000000000 ) ;
#2324=CARTESIAN_POINT ( 'NONE',  ( -25.00000000000000711, 53.00000000000000711, 0.5000000000000004441 ) ) ;
#2329=ORIENTED_EDGE ( 'NONE', *, *, #4305, .F. ) ;
#2340=CARTESIAN_POINT ( 'NONE',  ( -25.00000000000000000, 53.00000000000000711, -18.00000000000000355 ) ) ;
#2346=DIRECTION ( 'NONE',  ( 0.000000000000000000, 0.000000000000000000, -1.000000000000000000 ) ) ;
#2349=CARTESIAN_POINT ( 'NONE',  ( -41.00000000000000711, 110.0000000000000000, -5.000000000000000888 ) ) ;
#2354=LINE ( 'NONE', #10162, #338 ) ;
#2356=DIRECTION ( 'NONE',  ( 0.000000000000000000, 0.000000000000000000, -1.000000000000000000 ) ) ;
#2357=CARTESIAN_POINT ( 'NONE',  ( -24.00000000000000711, 53.00000000000000711, -30.99999999999999645 ) ) ;
#2358=VERTEX_POINT ( 'NONE', #11024 ) ;
#2381=VECTOR ( 'NONE', #19358, 1000.000000000000000 ) ;
#2398=EDGE_CURVE ( 'NONE', #18807, #19283, #18591, .T. ) ;
#2404=EDGE_CURVE ( 'NONE', #4659, #7333, #6343, .T. ) ;
#2407=EDGE_LOOP ( 'NONE', ( #11715, #12132, #2937, #4843 ) ) ;
#2414=EDGE_CURVE ( 'NONE', #15895, #11533, #15638, .T. ) ;
#2420=PRESENTATION_STYLE_ASSIGNMENT (( #5189 ) ) ;
#2423=ORIENTED_EDGE ( 'NONE', *, *, #14694, .F. ) ;
#2428=CARTESIAN_POINT ( 'NONE',  ( -41.00000000000000711, 53.00000000000000711, -38.50000000000000711 ) ) ;
#2439=EDGE_CURVE ( 'NONE', #7469, #17238, #5158, .T. ) ;
#2442=CARTESIAN_POINT ( 'NONE',  ( -41.00000000000000711, 110.0000000000000000, -30.99999999999999645 ) ) ;
#2444=ORIENTED_EDGE ( 'NONE', *, *, #7937, .F. ) ;
#2445=ORIENTED_EDGE ( 'NONE', *, *, #17190, .T. ) ;
#2448=DIRECTION ( 'NONE',  ( 0.000000000000000000, 0.000000000000000000, -1.000000000000000000 ) ) ;
#2449=ORIENTED_EDGE ( 'NONE', *, *, #5921, .T. ) ;
#2452=EDGE_CURVE ( 'NONE', #4121, #15591, #10734, .T. ) ;
#2456=CARTESIAN_POINT ( 'NONE',  ( -41.00000000000000711, 53.00000000000000711, -5.000000000000000888 ) ) ;
#2458=LINE ( 'NONE', #8631, #14071 ) ;
#2459=ORIENTED_EDGE ( 'NONE', *, *, #19083, .F. ) ;
#2460=CARTESIAN_POINT ( 'NONE',  ( -25.00000000000000000, 110.0000000000000000, 30.00000000000000000 ) ) ;
#2463=CARTESIAN_POINT ( 'NONE',  ( -41.00000000000000711, 53.00000000000000711, 20.00000000000000000 ) ) ;
#2465=DIRECTION ( 'NONE',  ( 0.000000000000000000, -1.000000000000000000, -0.000000000000000000 ) ) ;
#2486=VECTOR ( 'NONE', #13156, 1000.000000000000000 ) ;
#2488=CARTESIAN_POINT ( 'NONE',  ( -41.00000000000000711, 110.0000000000000000, 21.00000000000000000 ) ) ;
#2492=EDGE_CURVE ( 'NONE', #12636, #14875, #9834, .T. ) ;
#2497=LINE ( 'NONE', #8484, #1310 ) ;
#2512=CARTESIAN_POINT ( 'NONE',  ( -41.00000000000000711, 110.0000000000000000, 1.500000000000001332 ) ) ;
#2524=FACE_OUTER_BOUND ( 'NONE', #13829, .T. ) ;
#2527=ORIENTED_EDGE ( 'NONE', *, *, #2452, .T. ) ;
#2529=VECTOR ( 'NONE', #8495, 1000.000000000000000 ) ;
#2531=ORIENTED_EDGE ( 'NONE', *, *, #8652, .T. ) ;
#2540=FACE_OUTER_BOUND ( 'NONE', #8912, .T. ) ;
#2547=CARTESIAN_POINT ( 'NONE',  ( -41.00000000000000711, 53.00000000000000711, 26.50000000000000000 ) ) ;
#2566=DIRECTION ( 'NONE',  ( 1.000000000000000000, 1.156482317317871725E-16, -0.000000000000000000 ) ) ;
#2569=EDGE_CURVE ( 'NONE', #18998, #18134, #17590, .T. ) ;
#2574=EDGE_CURVE ( 'NONE', #4107, #4659, #7190, .T. ) ;
#2581=CARTESIAN_POINT ( 'NONE',  ( -41.00000000000000711, 53.00000000000000711, 26.50000000000000000 ) ) ;
#2582=CARTESIAN_POINT ( 'NONE',  ( -40.00000000000000711, 110.0000000000000000, -19.00000000000000355 ) ) ;
#2587=CARTESIAN_POINT ( 'NONE',  ( -32.50000000000000000, 53.00000000000000711, 15.00000000000000000 ) ) ;
#2590=VERTEX_POINT ( 'NONE', #4167 ) ;
#2603=DIRECTION ( 'NONE',  ( 0.000000000000000000, 0.000000000000000000, 1.000000000000000000 ) ) ;
#2605=CARTESIAN_POINT ( 'NONE',  ( -40.00000000000000711, 110.0000000000000000, 30.00000000000000000 ) ) ;
#2609=VERTEX_POINT ( 'NONE', #17007 ) ;
#2619=EDGE_LOOP ( 'NONE', ( #13810, #16935, #15387, #13295 ) ) ;
#2620=AXIS2_PLACEMENT_3D ( 'NONE', #809, #2566, #7074 ) ;
#2621=DIRECTION ( 'NONE',  ( -0.000000000000000000, -0.000000000000000000, -1.000000000000000000 ) ) ;
#2624=LINE ( 'NONE', #2349, #10921 ) ;
#2625=CARTESIAN_POINT ( 'NONE',  ( -41.00000000000000711, 53.00000000000000711, -30.99999999999999645 ) ) ;
#2632=EDGE_LOOP ( 'NONE', ( #9083, #4504, #1768, #9775 ) ) ;
#2637=DIRECTION ( 'NONE',  ( 0.000000000000000000, -1.000000000000000000, 0.000000000000000000 ) ) ;
#2638=ORIENTED_EDGE ( 'NONE', *, *, #16555, .F. ) ;
#2647=ORIENTED_EDGE ( 'NONE', *, *, #8995, .F. ) ;
#2649=ORIENTED_EDGE ( 'NONE', *, *, #17189, .T. ) ;
#2651=DIRECTION ( 'NONE',  ( -0.000000000000000000, -0.000000000000000000, -1.000000000000000000 ) ) ;
#2656=DIRECTION ( 'NONE',  ( -1.000000000000000000, 0.000000000000000000, -0.000000000000000000 ) ) ;
#2659=FACE_BOUND ( 'NONE', #11637, .T. ) ;
#2673=DIRECTION ( 'NONE',  ( 0.000000000000000000, 0.000000000000000000, -1.000000000000000000 ) ) ;
#2677=EDGE_CURVE ( 'NONE', #19215, #11338, #6321, .T. ) ;
#2685=PRODUCT_DEFINITION_SHAPE ( 'NONE', 'NONE',  #9182 ) ;
#2687=EDGE_CURVE ( 'NONE', #16539, #2590, #5044, .T. ) ;
#2698=EDGE_CURVE ( 'NONE', #15286, #14415, #16572, .T. ) ;
#2700=LINE ( 'NONE', #10432, #10637 ) ;
#2707=( GEOMETRIC_REPRESENTATION_CONTEXT ( 3 ) GLOBAL_UNCERTAINTY_ASSIGNED_CONTEXT ( ( #16714 ) ) GLOBAL_UNIT_ASSIGNED_CONTEXT ( ( #12339, #6186, #18241 ) ) REPRESENTATION_CONTEXT ( 'NONE', 'WORKASPACE' ) );
#2708=VECTOR ( 'NONE', #14350, 1000.000000000000000 ) ;
#2722=CARTESIAN_POINT ( 'NONE',  ( -32.50000000000000000, 53.00000000000000711, 17.64999999999998437 ) ) ;
#2727=ORIENTED_EDGE ( 'NONE', *, *, #7372, .T. ) ;
#2737=ORIENTED_EDGE ( 'NONE', *, *, #8879, .T. ) ;
#2742=ORIENTED_EDGE ( 'NONE', *, *, #16837, .F. ) ;
#2748=ORIENTED_EDGE ( 'NONE', *, *, #7353, .T. ) ;
#2754=PLANE ( 'NONE',  #12879 ) ;
#2782=VECTOR ( 'NONE', #4479, 1000.000000000000000 ) ;
#2797=VECTOR ( 'NONE', #5397, 1000.000000000000000 ) ;
#2798=CARTESIAN_POINT ( 'NONE',  ( -41.00000000000000711, 110.0000000000000000, 1.500000000000001332 ) ) ;
#2807=ORIENTED_EDGE ( 'NONE', *, *, #9847, .T. ) ;
#2810=EDGE_CURVE ( 'NONE', #16642, #6640, #12148, .T. ) ;
#2813=ORIENTED_EDGE ( 'NONE', *, *, #2492, .F. ) ;
#2832=EDGE_CURVE ( 'NONE', #1370, #6673, #7755, .T. ) ;
#2835=VERTEX_POINT ( 'NONE', #17850 ) ;
#2837=DIRECTION ( 'NONE',  ( 0.000000000000000000, 0.000000000000000000, -1.000000000000000000 ) ) ;
#2843=CARTESIAN_POINT ( 'NONE',  ( -24.00000000000000000, 53.00000000000000711, 21.00000000000000000 ) ) ;
#2844=ADVANCED_FACE ( 'NONE', ( #3041 ), #10679, .F. ) ;
#2854=FACE_OUTER_BOUND ( 'NONE', #12466, .T. ) ;
#2857=DIRECTION ( 'NONE',  ( -1.156482317317871478E-16, 1.000000000000000000, 0.000000000000000000 ) ) ;
#2863=ORIENTED_EDGE ( 'NONE', *, *, #8533, .T. ) ;
#2871=EDGE_LOOP ( 'NONE', ( #6456, #5564, #15323, #12070 ) ) ;
#2873=ORIENTED_EDGE ( 'NONE', *, *, #14905, .T. ) ;
#2876=LINE ( 'NONE', #2581, #2 ) ;
#2877=CARTESIAN_POINT ( 'NONE',  ( -41.00000000000000711, 110.0000000000000000, 20.00000000000000000 ) ) ;
#2881=FACE_BOUND ( 'NONE', #9818, .T. ) ;
#2886=EDGE_CURVE ( 'NONE', #13949, #5657, #9117, .T. ) ;
#2900=CARTESIAN_POINT ( 'NONE',  ( -40.00000000000000000, 53.00000000000000711, 30.00000000000000000 ) ) ;
#2906=PLANE ( 'NONE',  #10182 ) ;
#2907=ORIENTED_EDGE ( 'NONE', *, *, #12486, .F. ) ;
#2910=LINE ( 'NONE', #5956, #15679 ) ;
#2911=VERTEX_POINT ( 'NONE', #2059 ) ;
#2919=ORIENTED_EDGE ( 'NONE', *, *, #1250, .F. ) ;
#2925=CARTESIAN_POINT ( 'NONE',  ( -40.00000000000000000, 53.00000000000000711, 0.5000000000000004441 ) ) ;
#2931=VERTEX_POINT ( 'NONE', #7854 ) ;
#2937=ORIENTED_EDGE ( 'NONE', *, *, #659, .F. ) ;
#2941=DIRECTION ( 'NONE',  ( 0.000000000000000000, 0.000000000000000000, 1.000000000000000000 ) ) ;
#2944=CARTESIAN_POINT ( 'NONE',  ( -40.00000000000000711, 113.0000000000000000, -45.00000000000000000 ) ) ;
#2955=MECHANICAL_DESIGN_GEOMETRIC_PRESENTATION_REPRESENTATION('',(#14850),#2008);
#2956=CARTESIAN_POINT ( 'NONE',  ( -41.00000000000000711, 53.00000000000000711, 14.50000000000000000 ) ) ;
#2959=ORIENTED_EDGE ( 'NONE', *, *, #11929, .F. ) ;
#2972=DIRECTION ( 'NONE',  ( 0.000000000000000000, -1.000000000000000000, 0.000000000000000000 ) ) ;
#2980=VERTEX_POINT ( 'NONE', #3716 ) ;
#2991=VECTOR ( 'NONE', #11645, 1000.000000000000000 ) ;
#2993=CARTESIAN_POINT ( 'NONE',  ( -25.00000000000000711, 110.0000000000000000, 6.999999999999999112 ) ) ;
#2994=EDGE_CURVE ( 'NONE', #12352, #18999, #18441, .T. ) ;
#3017=VERTEX_POINT ( 'NONE', #5009 ) ;
#3018=LINE ( 'NONE', #13299, #18825 ) ;
#3022=DIRECTION ( 'NONE',  ( 0.000000000000000000, 1.000000000000000000, 0.000000000000000000 ) ) ;
#3023=ADVANCED_FACE ( 'NONE', ( #12254 ), #10968, .T. ) ;
#3027=CARTESIAN_POINT ( 'NONE',  ( -40.00000000000000711, 110.0000000000000000, 30.00000000000000000 ) ) ;
#3039=ADVANCED_FACE ( 'NONE', ( #9501 ), #11064, .T. ) ;
#3041=FACE_OUTER_BOUND ( 'NONE', #4414, .T. ) ;
#3042=EDGE_LOOP ( 'NONE', ( #2907, #7887, #6384, #15431 ) ) ;
#3048=ORIENTED_EDGE ( 'NONE', *, *, #16453, .F. ) ;
#3053=DIRECTION ( 'NONE',  ( -1.156482317317871478E-16, 1.000000000000000000, 0.000000000000000000 ) ) ;
#3055=DIRECTION ( 'NONE',  ( 0.000000000000000000, -1.000000000000000000, 0.000000000000000000 ) ) ;
#3070=CARTESIAN_POINT ( 'NONE',  ( -41.00000000000000711, 53.00000000000000711, -30.99999999999999645 ) ) ;
#3071=CARTESIAN_POINT ( 'NONE',  ( -25.00000000000000000, 113.0000000000000000, -50.00000000000000000 ) ) ;
#3089=LINE ( 'NONE', #17907, #18761 ) ;
#3096=LINE ( 'NONE', #927, #18665 ) ;
#3097=EDGE_CURVE ( 'NONE', #6553, #9106, #773, .T. ) ;
#3098=CARTESIAN_POINT ( 'NONE',  ( -40.00000000000000711, 110.0000000000000000, 14.50000000000000000 ) ) ;
#3101=EDGE_LOOP ( 'NONE', ( #19144, #17751, #13426, #18140 ) ) ;
#3103=VECTOR ( 'NONE', #8262, 1000.000000000000000 ) ;
#3106=EDGE_LOOP ( 'NONE', ( #14869, #7316, #14335, #3048 ) ) ;
#3107=ORIENTED_EDGE ( 'NONE', *, *, #16225, .T. ) ;
#3115=VERTEX_POINT ( 'NONE', #4102 ) ;
#3116=ORIENTED_EDGE ( 'NONE', *, *, #7505, .T. ) ;
#3117=LINE ( 'NONE', #7330, #977 ) ;
#3127=EDGE_LOOP ( 'NONE', ( #7341, #13695, #17840, #4878 ) ) ;
#3133=VECTOR ( 'NONE', #11633, 1000.000000000000000 ) ;
#3136=EDGE_CURVE ( 'NONE', #6673, #15600, #5474, .T. ) ;
#3139=CARTESIAN_POINT ( 'NONE',  ( -41.00000000000000711, 53.00000000000000711, -12.50000000000000000 ) ) ;
#3140=ORIENTED_EDGE ( 'NONE', *, *, #11983, .F. ) ;
#3148=DIRECTION ( 'NONE',  ( 0.000000000000000000, 0.000000000000000000, -1.000000000000000000 ) ) ;
#3150=AXIS2_PLACEMENT_3D ( 'NONE', #8537, #6969, #14324 ) ;
#3151=LINE ( 'NONE', #9515, #8966 ) ;
#3152=DIRECTION ( 'NONE',  ( 0.000000000000000000, -1.000000000000000000, 0.000000000000000000 ) ) ;
#3157=EDGE_CURVE ( 'NONE', #2911, #15600, #13100, .T. ) ;
#3167=DIRECTION ( 'NONE',  ( 0.000000000000000000, 0.000000000000000000, -1.000000000000000000 ) ) ;
#3171=VERTEX_POINT ( 'NONE', #2722 ) ;
#3173=LINE ( 'NONE', #11785, #472 ) ;
#3174=VECTOR ( 'NONE', #4385, 1000.000000000000000 ) ;
#3175=CARTESIAN_POINT ( 'NONE',  ( -24.00000000000000711, 53.00000000000000711, -44.00000000000000000 ) ) ;
#3178=ADVANCED_FACE ( 'NONE', ( #15776 ), #17337, .T. ) ;
#3179=CARTESIAN_POINT ( 'NONE',  ( -24.00000000000000000, 53.00000000000000711, -44.00000000000000000 ) ) ;
#3185=AXIS2_PLACEMENT_3D ( 'NONE', #8363, #2465, #5510 ) ;
#3195=DIRECTION ( 'NONE',  ( -0.000000000000000000, 1.000000000000000000, -0.000000000000000000 ) ) ;
#3201=VECTOR ( 'NONE', #9235, 1000.000000000000000 ) ;
#3202=DIRECTION ( 'NONE',  ( 1.000000000000000000, -0.000000000000000000, -0.000000000000000000 ) ) ;
#3205=CARTESIAN_POINT ( 'NONE',  ( -41.00000000000000711, 53.00000000000000711, -45.00000000000000000 ) ) ;
#3223=EDGE_LOOP ( 'NONE', ( #5305, #12286, #13981, #2245 ) ) ;
#3231=ORIENTED_EDGE ( 'NONE', *, *, #16480, .F. ) ;
#3235=ORIENTED_EDGE ( 'NONE', *, *, #4338, .F. ) ;
#3240=CARTESIAN_POINT ( 'NONE',  ( -41.00000000000000711, 53.00000000000000711, 6.999999999999999112 ) ) ;
#3252=PLANE ( 'NONE',  #8645 ) ;
#3254=ADVANCED_FACE ( 'NONE', ( #19004 ), #6757, .T. ) ;
#3261=LINE ( 'NONE', #9232, #17730 ) ;
#3264=EDGE_CURVE ( 'NONE', #16948, #4790, #17040, .T. ) ;
#3293=CARTESIAN_POINT ( 'NONE',  ( -24.00000000000000000, 110.0000000000000000, 30.00000000000000000 ) ) ;
#3296=LINE ( 'NONE', #4672, #9754 ) ;
#3301=VECTOR ( 'NONE', #12288, 1000.000000000000000 ) ;
#3306=EDGE_LOOP ( 'NONE', ( #5461, #1780, #9762, #9494 ) ) ;
#3315=VECTOR ( 'NONE', #19336, 1000.000000000000000 ) ;
#3316=AXIS2_PLACEMENT_3D ( 'NONE', #5169, #8214, #5082 ) ;
#3325=DIRECTION ( 'NONE',  ( -1.000000000000000000, 0.000000000000000000, -0.000000000000000000 ) ) ;
#3326=LINE ( 'NONE', #13701, #4435 ) ;
#3327=APPLICATION_CONTEXT ( 'automotive_design' ) ;
#3328=DIRECTION ( 'NONE',  ( 0.000000000000000000, -1.000000000000000000, 0.000000000000000000 ) ) ;
#3334=ORIENTED_EDGE ( 'NONE', *, *, #5808, .T. ) ;
#3342=CARTESIAN_POINT ( 'NONE',  ( -41.00000000000000711, 110.0000000000000000, -24.49999999999999645 ) ) ;
#3347=VERTEX_POINT ( 'NONE', #12869 ) ;
#3354=LINE ( 'NONE', #13927, #4875 ) ;
#3357=DIRECTION ( 'NONE',  ( 0.000000000000000000, 1.000000000000000000, 0.000000000000000000 ) ) ;
#3363=LINE ( 'NONE', #3645, #529 ) ;
#3367=ORIENTED_EDGE ( 'NONE', *, *, #4746, .T. ) ;
#3368=DIRECTION ( 'NONE',  ( -1.000000000000000000, 0.000000000000000000, -0.000000000000000000 ) ) ;
#3372=CARTESIAN_POINT ( 'NONE',  ( -41.00000000000000711, 110.0000000000000000, -5.000000000000004441 ) ) ;
#3381=EDGE_CURVE ( 'NONE', #18025, #17238, #913, .T. ) ;
#3385=DIRECTION ( 'NONE',  ( -1.000000000000000000, 0.000000000000000000, -0.000000000000000000 ) ) ;
#3390=DIRECTION ( 'NONE',  ( 1.000000000000000000, -0.000000000000000000, -0.000000000000000000 ) ) ;
#3391=LINE ( 'NONE', #9362, #836 ) ;
#3395=EDGE_CURVE ( 'NONE', #9366, #7944, #9917, .T. ) ;
#3396=EDGE_CURVE ( 'NONE', #7331, #4488, #6019, .T. ) ;
#3399=ADVANCED_FACE ( 'NONE', ( #16399 ), #5816, .F. ) ;
#3404=CARTESIAN_POINT ( 'NONE',  ( -41.00000000000000711, 110.0000000000000000, -12.50000000000000000 ) ) ;
#3410=AXIS2_PLACEMENT_3D ( 'NONE', #4278, #11806, #1335 ) ;
#3414=CARTESIAN_POINT ( 'NONE',  ( -40.00000000000000711, 53.00000000000000711, 21.00000000000000000 ) ) ;
#3416=CARTESIAN_POINT ( 'NONE',  ( -25.00000000000000000, 53.00000000000000711, -12.49999999999999645 ) ) ;
#3436=ORIENTED_EDGE ( 'NONE', *, *, #1878, .T. ) ;
#3442=PLANE ( 'NONE',  #6856 ) ;
#3445=CARTESIAN_POINT ( 'NONE',  ( -25.00000000000000711, 53.00000000000000711, 8.000000000000000000 ) ) ;
#3449=DIRECTION ( 'NONE',  ( -1.156482317317871478E-16, 1.000000000000000000, 0.000000000000000000 ) ) ;
#3458=EDGE_CURVE ( 'NONE', #10251, #10640, #17772, .T. ) ;
#3461=LINE ( 'NONE', #18569, #941 ) ;
#3464=LINE ( 'NONE', #12378, #9375 ) ;
#3465=ORIENTED_EDGE ( 'NONE', *, *, #7972, .F. ) ;
#3470=EDGE_CURVE ( 'NONE', #982, #17652, #9398, .T. ) ;
#3484=DIRECTION ( 'NONE',  ( -1.156482317317871478E-16, 1.000000000000000000, 0.000000000000000000 ) ) ;
#3489=DIRECTION ( 'NONE',  ( 0.000000000000000000, 0.000000000000000000, -1.000000000000000000 ) ) ;
#3492=LINE ( 'NONE', #9466, #2708 ) ;
#3494=EDGE_CURVE ( 'NONE', #2269, #15646, #4648, .T. ) ;
#3499=ORIENTED_EDGE ( 'NONE', *, *, #13062, .F. ) ;
#3504=ORIENTED_EDGE ( 'NONE', *, *, #9649, .T. ) ;
#3506=DIRECTION ( 'NONE',  ( 1.000000000000000000, -0.000000000000000000, -0.000000000000000000 ) ) ;
#3509=VECTOR ( 'NONE', #3053, 1000.000000000000000 ) ;
#3528=VERTEX_POINT ( 'NONE', #7474 ) ;
#3533=ORIENTED_EDGE ( 'NONE', *, *, #656, .T. ) ;
#3548=DIRECTION ( 'NONE',  ( -0.000000000000000000, 1.000000000000000000, -0.000000000000000000 ) ) ;
#3549=DIRECTION ( 'NONE',  ( 0.000000000000000000, -1.000000000000000000, 0.000000000000000000 ) ) ;
#3553=LINE ( 'NONE', #7774, #7402 ) ;
#3559=CARTESIAN_POINT ( 'NONE',  ( -41.00000000000000711, 110.0000000000000000, 27.50000000000000000 ) ) ;
#3562=DIRECTION ( 'NONE',  ( 0.000000000000000000, 0.000000000000000000, 1.000000000000000000 ) ) ;
#3571=EDGE_CURVE ( 'NONE', #4981, #12140, #3461, .T. ) ;
#3574=COLOUR_RGB ( '', 0.72549020, 0.75294118, 0.79215686) ;
#3575=DIRECTION ( 'NONE',  ( 0.000000000000000000, 0.000000000000000000, -1.000000000000000000 ) ) ;
#3587=CARTESIAN_POINT ( 'NONE',  ( -24.00000000000000000, 53.00000000000000711, -12.49999999999999645 ) ) ;
#3589=VECTOR ( 'NONE', #12199, 1000.000000000000000 ) ;
#3603=CARTESIAN_POINT ( 'NONE',  ( -41.00000000000000711, 110.0000000000000000, 21.00000000000000355 ) ) ;
#3608=CARTESIAN_POINT ( 'NONE',  ( -40.00000000000000711, 53.00000000000000711, -24.49999999999999645 ) ) ;
#3613=VERTEX_POINT ( 'NONE', #15518 ) ;
#3614=VERTEX_POINT ( 'NONE', #16894 ) ;
#3617=ORIENTED_EDGE ( 'NONE', *, *, #7860, .F. ) ;
#3626=ORIENTED_EDGE ( 'NONE', *, *, #18436, .T. ) ;
#3645=CARTESIAN_POINT ( 'NONE',  ( -41.00000000000000711, 53.00000000000000711, -6.000000000000001776 ) ) ;
#3646=EDGE_CURVE ( 'NONE', #4945, #17638, #12573, .T. ) ;
#3648=ADVANCED_FACE ( 'NONE', ( #1992 ), #9238, .F. ) ;
#3652=VECTOR ( 'NONE', #7075, 1000.000000000000000 ) ;
#3657=ORIENTED_EDGE ( 'NONE', *, *, #10824, .F. ) ;
#3667=LINE ( 'NONE', #4583, #12398 ) ;
#3681=CARTESIAN_POINT ( 'NONE',  ( -40.00000000000000711, 113.0000000000000000, -32.00000000000000000 ) ) ;
#3682=EDGE_CURVE ( 'NONE', #14586, #17642, #11183, .T. ) ;
#3683=DIRECTION ( 'NONE',  ( 0.000000000000000000, 0.000000000000000000, -1.000000000000000000 ) ) ;
#3697=CARTESIAN_POINT ( 'NONE',  ( -40.00000000000000000, 53.00000000000000711, -6.000000000000001776 ) ) ;
#3703=CARTESIAN_POINT ( 'NONE',  ( -24.00000000000000000, 52.00000000000000711, 30.00000000000000000 ) ) ;
#3704=VERTEX_POINT ( 'NONE', #11558 ) ;
#3716=CARTESIAN_POINT ( 'NONE',  ( -40.00000000000000711, 110.0000000000000000, 0.5000000000000004441 ) ) ;
#3720=ORIENTED_EDGE ( 'NONE', *, *, #15157, .T. ) ;
#3721=CARTESIAN_POINT ( 'NONE',  ( -24.00000000000000000, 53.00000000000000711, 30.00000000000000000 ) ) ;
#3733=ORIENTED_EDGE ( 'NONE', *, *, #2687, .T. ) ;
#3735=ADVANCED_FACE ( 'NONE', ( #14417 ), #2278, .T. ) ;
#3738=CARTESIAN_POINT ( 'NONE',  ( -41.00000000000000711, 53.00000000000000711, -32.00000000000000000 ) ) ;
#3739=ORIENTED_EDGE ( 'NONE', *, *, #6928, .T. ) ;
#3748=VECTOR ( 'NONE', #10264, 1000.000000000000000 ) ;
#3749=CARTESIAN_POINT ( 'NONE',  ( -41.00000000000000711, 53.00000000000000711, -45.00000000000000000 ) ) ;
#3751=DIRECTION ( 'NONE',  ( 0.000000000000000000, 0.000000000000000000, 1.000000000000000000 ) ) ;
#3752=LINE ( 'NONE', #5041, #10802 ) ;
#3754=EDGE_CURVE ( 'NONE', #2028, #10481, #5702, .T. ) ;
#3756=VECTOR ( 'NONE', #3751, 1000.000000000000000 ) ;
#3757=DIRECTION ( 'NONE',  ( 0.000000000000000000, -0.000000000000000000, 1.000000000000000000 ) ) ;
#3763=ORIENTED_EDGE ( 'NONE', *, *, #9077, .F. ) ;
#3771=CARTESIAN_POINT ( 'NONE',  ( -41.00000000000000711, 53.00000000000000711, 14.50000000000000000 ) ) ;
#3777=ADVANCED_FACE ( 'NONE', ( #11367 ), #17275, .T. ) ;
#3780=VECTOR ( 'NONE', #17971, 1000.000000000000000 ) ;
#3793=AXIS2_PLACEMENT_3D ( 'NONE', #2456, #8442, #3841 ) ;
#3796=VERTEX_POINT ( 'NONE', #1485 ) ;
#3799=VECTOR ( 'NONE', #6794, 1000.000000000000000 ) ;
#3806=ORIENTED_EDGE ( 'NONE', *, *, #4837, .T. ) ;
#3810=ORIENTED_EDGE ( 'NONE', *, *, #9670, .F. ) ;
#3814=VECTOR ( 'NONE', #17152, 1000.000000000000000 ) ;
#3820=ORIENTED_EDGE ( 'NONE', *, *, #18436, .F. ) ;
#3832=EDGE_LOOP ( 'NONE', ( #11545, #18861, #5494, #11294 ) ) ;
#3835=CARTESIAN_POINT ( 'NONE',  ( -24.00000000000000000, 110.0000000000000000, 30.00000000000000000 ) ) ;
#3837=VECTOR ( 'NONE', #16551, 1000.000000000000000 ) ;
#3841=DIRECTION ( 'NONE',  ( -1.000000000000000000, 0.000000000000000000, -0.000000000000000000 ) ) ;
#3842=VERTEX_POINT ( 'NONE', #5793 ) ;
#3843=DIRECTION ( 'NONE',  ( 0.000000000000000000, 0.000000000000000000, 1.000000000000000000 ) ) ;
#3847=EDGE_CURVE ( 'NONE', #7381, #12041, #17754, .T. ) ;
#3851=FACE_BOUND ( 'NONE', #7440, .T. ) ;
#3852=PLANE ( 'NONE',  #3185 ) ;
#3857=VERTEX_POINT ( 'NONE', #13531 ) ;
#3863=CARTESIAN_POINT ( 'NONE',  ( -41.00000000000000711, 53.00000000000000711, -19.00000000000000000 ) ) ;
#3871=DIRECTION ( 'NONE',  ( 1.000000000000000000, -0.000000000000000000, -0.000000000000000000 ) ) ;
#3873=EDGE_CURVE ( 'NONE', #4404, #17838, #6091, .T. ) ;
#3877=DIRECTION ( 'NONE',  ( -0.000000000000000000, 1.000000000000000000, -0.000000000000000000 ) ) ;
#3886=LINE ( 'NONE', #6827, #2150 ) ;
#3888=AXIS2_PLACEMENT_3D ( 'NONE', #17191, #5509, #3757 ) ;
#3896=SHAPE_REPRESENTATION_RELATIONSHIP ( 'NONE' , 'NONE' ,  #15908, #11089 ) ;
#3903=VECTOR ( 'NONE', #3484, 1000.000000000000000 ) ;
#3907=ORIENTED_EDGE ( 'NONE', *, *, #258, .T. ) ;
#3908=DIRECTION ( 'NONE',  ( 0.000000000000000000, 1.000000000000000000, 0.000000000000000000 ) ) ;
#3910=CARTESIAN_POINT ( 'NONE',  ( -25.00000000000000000, 53.00000000000000711, -25.49999999999999645 ) ) ;
#3918=CARTESIAN_POINT ( 'NONE',  ( -41.00000000000000711, 110.0000000000000000, 8.000000000000000000 ) ) ;
#3921=EDGE_CURVE ( 'NONE', #9405, #11598, #10183, .T. ) ;
#3925=LINE ( 'NONE', #11175, #1141 ) ;
#3928=CARTESIAN_POINT ( 'NONE',  ( -41.00000000000000711, 110.0000000000000000, -5.000000000000000888 ) ) ;
#3929=EDGE_LOOP ( 'NONE', ( #12447, #17364, #11251, #16552 ) ) ;
#3932=CARTESIAN_POINT ( 'NONE',  ( -41.00000000000000711, 110.0000000000000000, -44.00000000000000000 ) ) ;
#3943=PLANE ( 'NONE',  #2620 ) ;
#3944=EDGE_CURVE ( 'NONE', #14005, #13130, #8720, .T. ) ;
#3946=CARTESIAN_POINT ( 'NONE',  ( -25.00000000000000000, 53.00000000000000711, 30.00000000000000000 ) ) ;
#3949=EDGE_LOOP ( 'NONE', ( #9113, #7233, #1762, #2647 ) ) ;
#3951=UNCERTAINTY_MEASURE_WITH_UNIT (LENGTH_MEASURE( 1.000000000000000082E-05 ), #4036, 'distance_accuracy_value', 'NONE');
#3955=DIRECTION ( 'NONE',  ( 0.000000000000000000, -1.000000000000000000, 0.000000000000000000 ) ) ;
#3962=LINE ( 'NONE', #7093, #18137 ) ;
#3966=DIRECTION ( 'NONE',  ( 0.000000000000000000, 1.000000000000000000, 0.000000000000000000 ) ) ;
#3968=CARTESIAN_POINT ( 'NONE',  ( -25.00000000000000711, 110.0000000000000000, 13.50000000000000000 ) ) ;
#3972=EDGE_CURVE ( 'NONE', #1793, #9810, #14912, .T. ) ;
#3984=DIRECTION ( 'NONE',  ( 1.000000000000000000, -0.000000000000000000, -0.000000000000000000 ) ) ;
#3985=DIRECTION ( 'NONE',  ( 0.000000000000000000, 0.000000000000000000, -1.000000000000000000 ) ) ;
#3988=EDGE_CURVE ( 'NONE', #10297, #18278, #9600, .T. ) ;
#3989=FACE_OUTER_BOUND ( 'NONE', #15210, .T. ) ;
#4003=CARTESIAN_POINT ( 'NONE',  ( -41.00000000000000711, 110.0000000000000000, 21.00000000000000000 ) ) ;
#4004=ORIENTED_EDGE ( 'NONE', *, *, #2274, .T. ) ;
#4005=PLANE ( 'NONE',  #15346 ) ;
#4006=ORIENTED_EDGE ( 'NONE', *, *, #6514, .T. ) ;
#4018=VECTOR ( 'NONE', #6437, 1000.000000000000000 ) ;
#4030=CARTESIAN_POINT ( 'NONE',  ( -24.00000000000000000, 53.00000000000000711, 1.500000000000001332 ) ) ;
#4034=DIRECTION ( 'NONE',  ( 0.000000000000000000, 0.000000000000000000, 1.000000000000000000 ) ) ;
#4036=( LENGTH_UNIT ( ) NAMED_UNIT ( * ) SI_UNIT ( .MILLI., .METRE. ) );
#4037=EDGE_CURVE ( 'NONE', #12140, #7340, #13918, .T. ) ;
#4053=VECTOR ( 'NONE', #8211, 1000.000000000000000 ) ;
#4076=CARTESIAN_POINT ( 'NONE',  ( -40.00000000000000711, 113.0000000000000000, 30.00000000000000000 ) ) ;
#4083=VECTOR ( 'NONE', #7387, 1000.000000000000000 ) ;
#4084=CARTESIAN_POINT ( 'NONE',  ( -40.00000000000000711, 113.0000000000000000, 26.50000000000000000 ) ) ;
#4087=LINE ( 'NONE', #16434, #4902 ) ;
#4092=SURFACE_SIDE_STYLE ('',( #11337 ) ) ;
#4102=CARTESIAN_POINT ( 'NONE',  ( -41.00000000000000711, 53.00000000000000711, 13.50000000000000000 ) ) ;
#4105=VECTOR ( 'NONE', #9537, 1000.000000000000000 ) ;
#4107=VERTEX_POINT ( 'NONE', #19007 ) ;
#4108=CARTESIAN_POINT ( 'NONE',  ( -25.00000000000000711, 53.00000000000000711, 20.00000000000000000 ) ) ;
#4109=ORIENTED_EDGE ( 'NONE', *, *, #12877, .T. ) ;
#4118=DIRECTION ( 'NONE',  ( 1.000000000000000000, -0.000000000000000000, -0.000000000000000000 ) ) ;
#4121=VERTEX_POINT ( 'NONE', #17251 ) ;
#4126=FACE_OUTER_BOUND ( 'NONE', #4455, .T. ) ;
#4129=EDGE_CURVE ( 'NONE', #3115, #7331, #5204, .T. ) ;
#4131=LINE ( 'NONE', #14230, #5012 ) ;
#4133=ADVANCED_FACE ( 'NONE', ( #968 ), #17524, .T. ) ;
#4139=PLANE ( 'NONE',  #5970 ) ;
#4140=EDGE_CURVE ( 'NONE', #2146, #10091, #14210, .T. ) ;
#4147=CARTESIAN_POINT ( 'NONE',  ( -24.00000000000000711, 110.0000000000000000, -18.00000000000000000 ) ) ;
#4158=ORIENTED_EDGE ( 'NONE', *, *, #3847, .F. ) ;
#4159=CARTESIAN_POINT ( 'NONE',  ( -25.00000000000000000, 110.0000000000000000, 30.00000000000000000 ) ) ;
#4161=FACE_OUTER_BOUND ( 'NONE', #14898, .T. ) ;
#4167=CARTESIAN_POINT ( 'NONE',  ( -40.00000000000000711, 53.00000000000000711, -37.50000000000000711 ) ) ;
#4171=EDGE_CURVE ( 'NONE', #12791, #15600, #6945, .T. ) ;
#4172=ORIENTED_EDGE ( 'NONE', *, *, #3494, .T. ) ;
#4199=DIRECTION ( 'NONE',  ( 0.000000000000000000, 0.000000000000000000, -1.000000000000000000 ) ) ;
#4217=CARTESIAN_POINT ( 'NONE',  ( -25.00000000000000711, 53.00000000000000711, -12.50000000000000000 ) ) ;
#4224=VERTEX_POINT ( 'NONE', #14299 ) ;
#4236=ADVANCED_FACE ( 'NONE', ( #6760 ), #868, .T. ) ;
#4243=ORIENTED_EDGE ( 'NONE', *, *, #9244, .F. ) ;
#4254=CARTESIAN_POINT ( 'NONE',  ( -25.00000000000000000, 110.0000000000000000, 21.00000000000000355 ) ) ;
#4255=CARTESIAN_POINT ( 'NONE',  ( -41.00000000000000711, 110.0000000000000000, -38.50000000000000711 ) ) ;
#4256=FACE_OUTER_BOUND ( 'NONE', #14275, .T. ) ;
#4261=AXIS2_PLACEMENT_3D ( 'NONE', #2512, #18531, #5099 ) ;
#4278=CARTESIAN_POINT ( 'NONE',  ( -41.00000000000000711, 110.0000000000000000, -11.50000000000000000 ) ) ;
#4285=AXIS2_PLACEMENT_3D ( 'NONE', #12655, #2448, #8259 ) ;
#4289=EDGE_CURVE ( 'NONE', #12847, #17825, #1258, .T. ) ;
#4300=ORIENTED_EDGE ( 'NONE', *, *, #1400, .T. ) ;
#4302=ORIENTED_EDGE ( 'NONE', *, *, #8741, .T. ) ;
#4303=ORIENTED_EDGE ( 'NONE', *, *, #10257, .T. ) ;
#4305=EDGE_CURVE ( 'NONE', #18807, #18025, #3117, .T. ) ;
#4306=DIRECTION ( 'NONE',  ( 1.000000000000000000, -0.000000000000000000, -0.000000000000000000 ) ) ;
#4307=LINE ( 'NONE', #7335, #7177 ) ;
#4309=DIRECTION ( 'NONE',  ( 0.000000000000000000, 0.000000000000000000, -1.000000000000000000 ) ) ;
#4313=ORIENTED_EDGE ( 'NONE', *, *, #2810, .T. ) ;
#4321=DIRECTION ( 'NONE',  ( 0.000000000000000000, -1.000000000000000000, 0.000000000000000000 ) ) ;
#4328=DIRECTION ( 'NONE',  ( 0.000000000000000000, 0.000000000000000000, -1.000000000000000000 ) ) ;
#4330=DIRECTION ( 'NONE',  ( 1.000000000000000000, 0.000000000000000000, 0.000000000000000000 ) ) ;
#4338=EDGE_CURVE ( 'NONE', #4981, #8044, #3018, .T. ) ;
#4340=ORIENTED_EDGE ( 'NONE', *, *, #18991, .T. ) ;
#4351=ORIENTED_EDGE ( 'NONE', *, *, #9053, .F. ) ;
#4376=VECTOR ( 'NONE', #3843, 1000.000000000000000 ) ;
#4378=AXIS2_PLACEMENT_3D ( 'NONE', #7043, #18823, #13012 ) ;
#4382=DIRECTION ( 'NONE',  ( 0.000000000000000000, 0.000000000000000000, -1.000000000000000000 ) ) ;
#4385=DIRECTION ( 'NONE',  ( 0.000000000000000000, -1.000000000000000000, 0.000000000000000000 ) ) ;
#4386=DIRECTION ( 'NONE',  ( 1.000000000000000000, -0.000000000000000000, -0.000000000000000000 ) ) ;
#4396=LINE ( 'NONE', #5960, #15216 ) ;
#4404=VERTEX_POINT ( 'NONE', #4803 ) ;
#4414=EDGE_LOOP ( 'NONE', ( #10066, #12931, #8487, #6214 ) ) ;
#4426=DIRECTION ( 'NONE',  ( 1.000000000000000000, -0.000000000000000000, -0.000000000000000000 ) ) ;
#4429=DIRECTION ( 'NONE',  ( 1.000000000000000000, -0.000000000000000000, -0.000000000000000000 ) ) ;
#4432=CARTESIAN_POINT ( 'NONE',  ( -24.00000000000000000, 53.00000000000000711, -45.00000000000000000 ) ) ;
#4435=VECTOR ( 'NONE', #15280, 1000.000000000000000 ) ;
#4443=ORIENTED_EDGE ( 'NONE', *, *, #3944, .T. ) ;
#4452=CARTESIAN_POINT ( 'NONE',  ( -25.00000000000000000, 53.00000000000000711, 6.999999999999999112 ) ) ;
#4455=EDGE_LOOP ( 'NONE', ( #8696, #7850, #17555, #2737 ) ) ;
#4457=EDGE_CURVE ( 'NONE', #12613, #6640, #10854, .T. ) ;
#4459=CARTESIAN_POINT ( 'NONE',  ( -40.00000000000000711, 113.0000000000000000, 30.00000000000000000 ) ) ;
#4461=DIRECTION ( 'NONE',  ( 0.000000000000000000, 0.000000000000000000, -1.000000000000000000 ) ) ;
#4466=DIRECTION ( 'NONE',  ( -0.000000000000000000, -0.000000000000000000, -1.000000000000000000 ) ) ;
#4478=DIRECTION ( 'NONE',  ( 0.000000000000000000, -1.000000000000000000, 0.000000000000000000 ) ) ;
#4479=DIRECTION ( 'NONE',  ( 1.156482317317871725E-16, -1.000000000000000000, 0.000000000000000000 ) ) ;
#4485=EDGE_CURVE ( 'NONE', #7631, #2980, #15375, .T. ) ;
#4488=VERTEX_POINT ( 'NONE', #6168 ) ;
#4501=ORIENTED_EDGE ( 'NONE', *, *, #16547, .T. ) ;
#4504=ORIENTED_EDGE ( 'NONE', *, *, #7119, .T. ) ;
#4508=EDGE_CURVE ( 'NONE', #14672, #1673, #564, .T. ) ;
#4521=DIRECTION ( 'NONE',  ( 0.000000000000000000, 0.000000000000000000, -1.000000000000000000 ) ) ;
#4528=ORIENTED_EDGE ( 'NONE', *, *, #132, .F. ) ;
#4529=DIRECTION ( 'NONE',  ( -1.000000000000000000, 0.000000000000000000, -0.000000000000000000 ) ) ;
#4532=DIRECTION ( 'NONE',  ( 0.000000000000000000, -1.000000000000000000, 0.000000000000000000 ) ) ;
#4534=SHAPE_DEFINITION_REPRESENTATION ( #2685, #15908 ) ;
#4548=VECTOR ( 'NONE', #11488, 1000.000000000000000 ) ;
#4549=LINE ( 'NONE', #10506, #15333 ) ;
#4553=PLANE ( 'NONE',  #11842 ) ;
#4554=EDGE_CURVE ( 'NONE', #11338, #12423, #9290, .T. ) ;
#4576=VECTOR ( 'NONE', #14401, 1000.000000000000000 ) ;
#4583=CARTESIAN_POINT ( 'NONE',  ( -41.00000000000000711, 53.00000000000000711, -24.49999999999999645 ) ) ;
#4592=ORIENTED_EDGE ( 'NONE', *, *, #4508, .T. ) ;
#4599=ORIENTED_EDGE ( 'NONE', *, *, #8394, .T. ) ;
#4610=VECTOR ( 'NONE', #3549, 1000.000000000000000 ) ;
#4625=ORIENTED_EDGE ( 'NONE', *, *, #7838, .T. ) ;
#4627=CARTESIAN_POINT ( 'NONE',  ( -40.00000000000000711, 110.0000000000000000, 30.00000000000000000 ) ) ;
#4628=VERTEX_POINT ( 'NONE', #6734 ) ;
#4637=DIRECTION ( 'NONE',  ( 1.000000000000000000, 0.000000000000000000, 0.000000000000000000 ) ) ;
#4645=EDGE_CURVE ( 'NONE', #1661, #3528, #18790, .T. ) ;
#4648=LINE ( 'NONE', #4452, #3780 ) ;
#4653=DIRECTION ( 'NONE',  ( 0.000000000000000000, 0.000000000000000000, -1.000000000000000000 ) ) ;
#4659=VERTEX_POINT ( 'NONE', #14091 ) ;
#4660=VECTOR ( 'NONE', #10338, 1000.000000000000000 ) ;
#4664=PLANE ( 'NONE',  #16335 ) ;
#4672=CARTESIAN_POINT ( 'NONE',  ( -25.00000000000000000, 53.00000000000000711, 30.00000000000000000 ) ) ;
#4678=FACE_OUTER_BOUND ( 'NONE', #16167, .T. ) ;
#4681=ORIENTED_EDGE ( 'NONE', *, *, #258, .F. ) ;
#4682=ORIENTED_EDGE ( 'NONE', *, *, #16091, .F. ) ;
#4691=AXIS2_PLACEMENT_3D ( 'NONE', #803, #9992, #9809 ) ;
#4699=CARTESIAN_POINT ( 'NONE',  ( -41.00000000000000711, 110.0000000000000000, 0.5000000000000004441 ) ) ;
#4703=CARTESIAN_POINT ( 'NONE',  ( -41.00000000000000711, 53.00000000000000711, -32.00000000000000000 ) ) ;
#4704=EDGE_CURVE ( 'NONE', #12989, #7863, #2318, .T. ) ;
#4709=VECTOR ( 'NONE', #7557, 1000.000000000000000 ) ;
#4712=ORIENTED_EDGE ( 'NONE', *, *, #6424, .T. ) ;
#4716=VECTOR ( 'NONE', #13153, 1000.000000000000000 ) ;
#4722=DIRECTION ( 'NONE',  ( 1.000000000000000000, -0.000000000000000000, -0.000000000000000000 ) ) ;
#4725=VECTOR ( 'NONE', #6268, 1000.000000000000000 ) ;
#4726=DIRECTION ( 'NONE',  ( 0.000000000000000000, 0.000000000000000000, 1.000000000000000000 ) ) ;
#4739=DIRECTION ( 'NONE',  ( 0.000000000000000000, 0.000000000000000000, -1.000000000000000000 ) ) ;
#4744=EDGE_CURVE ( 'NONE', #17457, #8804, #13376, .T. ) ;
#4746=EDGE_CURVE ( 'NONE', #17457, #12847, #2700, .T. ) ;
#4749=VECTOR ( 'NONE', #776, 1000.000000000000000 ) ;
#4751=EDGE_CURVE ( 'NONE', #14672, #19394, #2876, .T. ) ;
#4778=DIRECTION ( 'NONE',  ( 1.000000000000000000, -0.000000000000000000, -0.000000000000000000 ) ) ;
#4786=ADVANCED_FACE ( 'NONE', ( #10019 ), #5530, .T. ) ;
#4789=DIRECTION ( 'NONE',  ( -1.000000000000000000, 0.000000000000000000, -0.000000000000000000 ) ) ;
#4790=VERTEX_POINT ( 'NONE', #4459 ) ;
#4795=ORIENTED_EDGE ( 'NONE', *, *, #11894, .T. ) ;
#4802=ORIENTED_EDGE ( 'NONE', *, *, #13331, .T. ) ;
#4803=CARTESIAN_POINT ( 'NONE',  ( -40.00000000000000711, 110.0000000000000000, -5.000000000000000888 ) ) ;
#4810=CARTESIAN_POINT ( 'NONE',  ( -40.00000000000000711, 110.0000000000000000, -18.00000000000000000 ) ) ;
#4811=ORIENTED_EDGE ( 'NONE', *, *, #12644, .T. ) ;
#4813=ORIENTED_EDGE ( 'NONE', *, *, #2203, .F. ) ;
#4815=DIRECTION ( 'NONE',  ( 0.000000000000000000, 0.000000000000000000, 1.000000000000000000 ) ) ;
#4821=DIRECTION ( 'NONE',  ( 1.000000000000000000, -0.000000000000000000, -0.000000000000000000 ) ) ;
#4822=EDGE_LOOP ( 'NONE', ( #13936, #10362, #605, #12277 ) ) ;
#4824=ORIENTED_EDGE ( 'NONE', *, *, #3381, .F. ) ;
#4830=DIRECTION ( 'NONE',  ( -1.000000000000000000, -0.000000000000000000, 0.000000000000000000 ) ) ;
#4833=CARTESIAN_POINT ( 'NONE',  ( -24.00000000000000711, 110.0000000000000000, -37.50000000000000711 ) ) ;
#4836=ORIENTED_EDGE ( 'NONE', *, *, #8898, .F. ) ;
#4837=EDGE_CURVE ( 'NONE', #993, #7955, #17778, .T. ) ;
#4840=ORIENTED_EDGE ( 'NONE', *, *, #13917, .F. ) ;
#4843=ORIENTED_EDGE ( 'NONE', *, *, #13435, .T. ) ;
#4848=CARTESIAN_POINT ( 'NONE',  ( -40.00000000000000711, 113.0000000000000000, -6.000000000000005329 ) ) ;
#4870=ADVANCED_FACE ( 'NONE', ( #6994 ), #16110, .F. ) ;
#4875=VECTOR ( 'NONE', #8062, 1000.000000000000000 ) ;
#4878=ORIENTED_EDGE ( 'NONE', *, *, #13459, .F. ) ;
#4902=VECTOR ( 'NONE', #1143, 1000.000000000000000 ) ;
#4903=VECTOR ( 'NONE', #8861, 1000.000000000000000 ) ;
#4905=ORIENTED_EDGE ( 'NONE', *, *, #7714, .T. ) ;
#4920=ORIENTED_EDGE ( 'NONE', *, *, #9760, .F. ) ;
#4932=CARTESIAN_POINT ( 'NONE',  ( -41.00000000000000711, 53.00000000000000711, -5.000000000000000888 ) ) ;
#4944=LINE ( 'NONE', #17091, #7502 ) ;
#4945=VERTEX_POINT ( 'NONE', #8750 ) ;
#4976=ORIENTED_EDGE ( 'NONE', *, *, #3157, .T. ) ;
#4981=VERTEX_POINT ( 'NONE', #13832 ) ;
#4988=ORIENTED_EDGE ( 'NONE', *, *, #9738, .F. ) ;
#4998=CARTESIAN_POINT ( 'NONE',  ( -40.00000000000000711, 110.0000000000000000, -5.999999999999998224 ) ) ;
#5003=ORIENTED_EDGE ( 'NONE', *, *, #4457, .T. ) ;
#5009=CARTESIAN_POINT ( 'NONE',  ( -40.00000000000000711, 110.0000000000000000, 27.50000000000000000 ) ) ;
#5012=VECTOR ( 'NONE', #9716, 1000.000000000000000 ) ;
#5020=FACE_BOUND ( 'NONE', #1059, .T. ) ;
#5021=VECTOR ( 'NONE', #8372, 1000.000000000000000 ) ;
#5034=AXIS2_PLACEMENT_3D ( 'NONE', #2158, #2346, #14303 ) ;
#5036=CARTESIAN_POINT ( 'NONE',  ( -24.00000000000000000, 110.0000000000000000, 30.00000000000000000 ) ) ;
#5037=ORIENTED_EDGE ( 'NONE', *, *, #3847, .T. ) ;
#5038=DIRECTION ( 'NONE',  ( -0.000000000000000000, 1.000000000000000000, 0.000000000000000000 ) ) ;
#5041=CARTESIAN_POINT ( 'NONE',  ( -41.00000000000000711, 53.00000000000000711, 14.50000000000000000 ) ) ;
#5044=LINE ( 'NONE', #7892, #8451 ) ;
#5049=VECTOR ( 'NONE', #8, 1000.000000000000000 ) ;
#5056=ADVANCED_FACE ( 'NONE', ( #16982 ), #1879, .T. ) ;
#5069=CARTESIAN_POINT ( 'NONE',  ( -24.00000000000000711, 110.0000000000000000, -11.50000000000000000 ) ) ;
#5070=VECTOR ( 'NONE', #14961, 1000.000000000000000 ) ;
#5082=DIRECTION ( 'NONE',  ( -1.000000000000000000, 0.000000000000000000, -0.000000000000000000 ) ) ;
#5084=AXIS2_PLACEMENT_3D ( 'NONE', #6005, #13634, #11967 ) ;
#5087=ORIENTED_EDGE ( 'NONE', *, *, #14302, .F. ) ;
#5089=AXIS2_PLACEMENT_3D ( 'NONE', #17314, #3877, #17492 ) ;
#5091=LINE ( 'NONE', #10855, #17006 ) ;
#5097=LINE ( 'NONE', #3416, #12235 ) ;
#5099=DIRECTION ( 'NONE',  ( 0.000000000000000000, 0.000000000000000000, -1.000000000000000000 ) ) ;
#5101=ORIENTED_EDGE ( 'NONE', *, *, #11513, .T. ) ;
#5108=VECTOR ( 'NONE', #1752, 1000.000000000000000 ) ;
#5115=ORIENTED_EDGE ( 'NONE', *, *, #13054, .T. ) ;
#5116=CARTESIAN_POINT ( 'NONE',  ( -24.00000000000000711, 53.00000000000000711, 27.50000000000000000 ) ) ;
#5120=ADVANCED_FACE ( 'NONE', ( #18822 ), #5396, .T. ) ;
#5121=CARTESIAN_POINT ( 'NONE',  ( -41.00000000000000711, 110.0000000000000000, 8.000000000000000000 ) ) ;
#5122=FACE_OUTER_BOUND ( 'NONE', #13588, .T. ) ;
#5123=FACE_BOUND ( 'NONE', #11926, .T. ) ;
#5127=CARTESIAN_POINT ( 'NONE',  ( -41.00000000000000711, 110.0000000000000000, -38.50000000000000711 ) ) ;
#5133=ORIENTED_EDGE ( 'NONE', *, *, #6964, .F. ) ;
#5136=ORIENTED_EDGE ( 'NONE', *, *, #436, .F. ) ;
#5138=ORIENTED_EDGE ( 'NONE', *, *, #17086, .F. ) ;
#5142=LINE ( 'NONE', #8082, #14129 ) ;
#5146=ORIENTED_EDGE ( 'NONE', *, *, #10597, .F. ) ;
#5158=LINE ( 'NONE', #13876, #12473 ) ;
#5169=CARTESIAN_POINT ( 'NONE',  ( -41.00000000000000711, 53.00000000000000711, -24.49999999999999645 ) ) ;
#5180=EDGE_CURVE ( 'NONE', #7475, #13902, #2624, .T. ) ;
#5183=LINE ( 'NONE', #17139, #1281 ) ;
#5189=SURFACE_STYLE_USAGE ( .BOTH. , #4092 ) ;
#5203=EDGE_CURVE ( 'NONE', #3614, #1662, #14592, .T. ) ;
#5204=LINE ( 'NONE', #14390, #11593 ) ;
#5210=FACE_OUTER_BOUND ( 'NONE', #3101, .T. ) ;
#5213=VECTOR ( 'NONE', #4466, 1000.000000000000000 ) ;
#5216=DIRECTION ( 'NONE',  ( -1.000000000000000000, 0.000000000000000000, -0.000000000000000000 ) ) ;
#5218=EDGE_LOOP ( 'NONE', ( #130, #3334, #1580, #15814 ) ) ;
#5226=AXIS2_PLACEMENT_3D ( 'NONE', #18593, #3683, #2019 ) ;
#5230=VERTEX_POINT ( 'NONE', #16063 ) ;
#5235=DIRECTION ( 'NONE',  ( 0.000000000000000000, 0.000000000000000000, -1.000000000000000000 ) ) ;
#5243=EDGE_LOOP ( 'NONE', ( #4302, #11093, #10680, #16355 ) ) ;
#5248=CARTESIAN_POINT ( 'NONE',  ( -41.00000000000000711, 110.0000000000000000, 14.50000000000000000 ) ) ;
#5258=LINE ( 'NONE', #12692, #12700 ) ;
#5274=ORIENTED_EDGE ( 'NONE', *, *, #16091, .T. ) ;
#5295=FACE_BOUND ( 'NONE', #13993, .T. ) ;
#5296=EDGE_CURVE ( 'NONE', #11714, #12973, #8806, .T. ) ;
#5300=DIRECTION ( 'NONE',  ( 0.000000000000000000, 0.000000000000000000, -1.000000000000000000 ) ) ;
#5301=VECTOR ( 'NONE', #12684, 1000.000000000000000 ) ;
#5305=ORIENTED_EDGE ( 'NONE', *, *, #13190, .F. ) ;
#5308=ORIENTED_EDGE ( 'NONE', *, *, #8762, .T. ) ;
#5313=AXIS2_PLACEMENT_3D ( 'NONE', #6411, #1799, #3368 ) ;
#5323=VECTOR ( 'NONE', #9994, 1000.000000000000000 ) ;
#5326=SURFACE_SIDE_STYLE ('',( #14331 ) ) ;
#5331=DIRECTION ( 'NONE',  ( -1.000000000000000000, 0.000000000000000000, -0.000000000000000000 ) ) ;
#5342=VECTOR ( 'NONE', #6591, 1000.000000000000000 ) ;
#5343=CARTESIAN_POINT ( 'NONE',  ( -41.00000000000000711, 53.00000000000000711, 0.5000000000000004441 ) ) ;
#5352=DIRECTION ( 'NONE',  ( 0.000000000000000000, -1.000000000000000000, 0.000000000000000000 ) ) ;
#5353=VECTOR ( 'NONE', #14819, 1000.000000000000000 ) ;
#5360=DIRECTION ( 'NONE',  ( 0.000000000000000000, -1.000000000000000000, -0.000000000000000000 ) ) ;
#5367=VECTOR ( 'NONE', #9813, 1000.000000000000000 ) ;
#5382=ORIENTED_EDGE ( 'NONE', *, *, #14905, .F. ) ;
#5396=PLANE ( 'NONE',  #12789 ) ;
#5397=DIRECTION ( 'NONE',  ( -1.156482317317871478E-16, 1.000000000000000000, 0.000000000000000000 ) ) ;
#5422=PRESENTATION_STYLE_ASSIGNMENT (( #901 ) ) ;
#5461=ORIENTED_EDGE ( 'NONE', *, *, #12471, .F. ) ;
#5467=EDGE_CURVE ( 'NONE', #19215, #7148, #15379, .T. ) ;
#5471=AXIS2_PLACEMENT_3D ( 'NONE', #3863, #2673, #15822 ) ;
#5474=LINE ( 'NONE', #15962, #16603 ) ;
#5475=ORIENTED_EDGE ( 'NONE', *, *, #7103, .T. ) ;
#5482=DIRECTION ( 'NONE',  ( 0.000000000000000000, 0.000000000000000000, -1.000000000000000000 ) ) ;
#5490=ORIENTED_EDGE ( 'NONE', *, *, #4037, .T. ) ;
#5493=CARTESIAN_POINT ( 'NONE',  ( -40.00000000000000000, 53.00000000000000711, 6.999999999999999112 ) ) ;
#5494=ORIENTED_EDGE ( 'NONE', *, *, #8435, .T. ) ;
#5503=ORIENTED_EDGE ( 'NONE', *, *, #12877, .F. ) ;
#5506=LINE ( 'NONE', #1184, #17878 ) ;
#5509=DIRECTION ( 'NONE',  ( 0.000000000000000000, 1.000000000000000000, 0.000000000000000000 ) ) ;
#5510=DIRECTION ( 'NONE',  ( 0.000000000000000000, 0.000000000000000000, -1.000000000000000000 ) ) ;
#5512=VECTOR ( 'NONE', #4386, 1000.000000000000000 ) ;
#5514=ORIENTED_EDGE ( 'NONE', *, *, #19178, .T. ) ;
#5521=EDGE_CURVE ( 'NONE', #3347, #8366, #2320, .T. ) ;
#5528=CARTESIAN_POINT ( 'NONE',  ( -41.00000000000000711, 53.00000000000000711, 27.50000000000000000 ) ) ;
#5530=PLANE ( 'NONE',  #1260 ) ;
#5540=ORIENTED_EDGE ( 'NONE', *, *, #10084, .F. ) ;
#5542=( GEOMETRIC_REPRESENTATION_CONTEXT ( 3 ) GLOBAL_UNCERTAINTY_ASSIGNED_CONTEXT ( ( #15907 ) ) GLOBAL_UNIT_ASSIGNED_CONTEXT ( ( #14288, #6747, #18623 ) ) REPRESENTATION_CONTEXT ( 'NONE', 'WORKASPACE' ) );
#5557=EDGE_CURVE ( 'NONE', #7381, #16262, #16333, .T. ) ;
#5559=ORIENTED_EDGE ( 'NONE', *, *, #15157, .F. ) ;
#5564=ORIENTED_EDGE ( 'NONE', *, *, #5521, .F. ) ;
#5570=DIRECTION ( 'NONE',  ( 0.000000000000000000, 0.000000000000000000, -1.000000000000000000 ) ) ;
#5572=DIRECTION ( 'NONE',  ( 0.000000000000000000, 0.000000000000000000, -1.000000000000000000 ) ) ;
#5573=EDGE_LOOP ( 'NONE', ( #650, #12370, #14373, #12259 ) ) ;
#5575=ORIENTED_EDGE ( 'NONE', *, *, #11475, .T. ) ;
#5578=CARTESIAN_POINT ( 'NONE',  ( -40.00000000000000711, 113.0000000000000000, -50.00000000000000000 ) ) ;
#5585=ORIENTED_EDGE ( 'NONE', *, *, #625, .F. ) ;
#5586=ORIENTED_EDGE ( 'NONE', *, *, #19039, .F. ) ;
#5588=VECTOR ( 'NONE', #1337, 1000.000000000000000 ) ;
#5589=PLANE ( 'NONE',  #4285 ) ;
#5595=VECTOR ( 'NONE', #14276, 1000.000000000000000 ) ;
#5596=DIRECTION ( 'NONE',  ( 1.000000000000000000, -0.000000000000000000, -0.000000000000000000 ) ) ;
#5597=VERTEX_POINT ( 'NONE', #5846 ) ;
#5611=AXIS2_PLACEMENT_3D ( 'NONE', #3928, #17359, #15991 ) ;
#5613=VERTEX_POINT ( 'NONE', #17701 ) ;
#5615=VECTOR ( 'NONE', #5038, 1000.000000000000000 ) ;
#5621=ORIENTED_EDGE ( 'NONE', *, *, #876, .T. ) ;
#5626=DIRECTION ( 'NONE',  ( -0.000000000000000000, 1.000000000000000000, -0.000000000000000000 ) ) ;
#5634=DIRECTION ( 'NONE',  ( 0.000000000000000000, 0.000000000000000000, -1.000000000000000000 ) ) ;
#5642=EDGE_CURVE ( 'NONE', #7137, #5957, #19077, .T. ) ;
#5644=VECTOR ( 'NONE', #4309, 1000.000000000000000 ) ;
#5649=CARTESIAN_POINT ( 'NONE',  ( -41.00000000000000711, 53.00000000000000711, -44.00000000000000000 ) ) ;
#5653=CARTESIAN_POINT ( 'NONE',  ( -40.00000000000000711, 110.0000000000000000, 21.00000000000000000 ) ) ;
#5657=VERTEX_POINT ( 'NONE', #14858 ) ;
#5661=AXIS2_PLACEMENT_3D ( 'NONE', #4003, #691, #5572 ) ;
#5669=CARTESIAN_POINT ( 'NONE',  ( -24.00000000000000000, 53.00000000000000711, 20.00000000000000000 ) ) ;
#5677=DIRECTION ( 'NONE',  ( -0.000000000000000000, -0.000000000000000000, -1.000000000000000000 ) ) ;
#5685=DIRECTION ( 'NONE',  ( 1.156482317317871725E-16, -1.000000000000000000, 0.000000000000000000 ) ) ;
#5688=ORIENTED_EDGE ( 'NONE', *, *, #1106, .F. ) ;
#5693=VERTEX_POINT ( 'NONE', #11914 ) ;
#5702=LINE ( 'NONE', #3932, #17873 ) ;
#5706=DIRECTION ( 'NONE',  ( -1.000000000000000000, 0.000000000000000000, -0.000000000000000000 ) ) ;
#5713=DIRECTION ( 'NONE',  ( 0.000000000000000000, 0.000000000000000000, -1.000000000000000000 ) ) ;
#5715=DIRECTION ( 'NONE',  ( 0.000000000000000000, -1.000000000000000000, 0.000000000000000000 ) ) ;
#5716=ORIENTED_EDGE ( 'NONE', *, *, #2886, .T. ) ;
#5723=ORIENTED_EDGE ( 'NONE', *, *, #11548, .F. ) ;
#5730=EDGE_CURVE ( 'NONE', #4981, #2835, #16078, .T. ) ;
#5736=ORIENTED_EDGE ( 'NONE', *, *, #19064, .T. ) ;
#5766=ADVANCED_FACE ( 'NONE', ( #19026 ), #18840, .T. ) ;
#5780=ORIENTED_EDGE ( 'NONE', *, *, #18854, .T. ) ;
#5793=CARTESIAN_POINT ( 'NONE',  ( -41.00000000000000711, 110.0000000000000000, -19.00000000000000000 ) ) ;
#5797=FACE_OUTER_BOUND ( 'NONE', #14917, .T. ) ;
#5799=CARTESIAN_POINT ( 'NONE',  ( -41.00000000000000711, 53.00000000000000711, -38.50000000000000711 ) ) ;
#5802=FACE_OUTER_BOUND ( 'NONE', #7227, .T. ) ;
#5806=EDGE_CURVE ( 'NONE', #15519, #16834, #4131, .T. ) ;
#5808=EDGE_CURVE ( 'NONE', #16539, #2289, #798, .T. ) ;
#5816=PLANE ( 'NONE',  #6607 ) ;
#5822=CARTESIAN_POINT ( 'NONE',  ( -41.00000000000000711, 53.00000000000000711, -37.50000000000000711 ) ) ;
#5831=LINE ( 'NONE', #14746, #2323 ) ;
#5833=CARTESIAN_POINT ( 'NONE',  ( -41.00000000000000711, 110.0000000000000000, 14.50000000000000000 ) ) ;
#5846=CARTESIAN_POINT ( 'NONE',  ( -25.00000000000000711, 110.0000000000000000, 20.00000000000000000 ) ) ;
#5847=LINE ( 'NONE', #5944, #17791 ) ;
#5853=DIRECTION ( 'NONE',  ( 1.000000000000000000, -0.000000000000000000, -0.000000000000000000 ) ) ;
#5854=ORIENTED_EDGE ( 'NONE', *, *, #14798, .F. ) ;
#5855=ORIENTED_EDGE ( 'NONE', *, *, #12708, .F. ) ;
#5864=CARTESIAN_POINT ( 'NONE',  ( -25.00000000000000000, 113.0000000000000000, 30.00000000000000000 ) ) ;
#5870=ORIENTED_EDGE ( 'NONE', *, *, #15643, .F. ) ;
#5876=ORIENTED_EDGE ( 'NONE', *, *, #4751, .F. ) ;
#5886=EDGE_CURVE ( 'NONE', #14875, #10285, #3, .T. ) ;
#5904=CARTESIAN_POINT ( 'NONE',  ( -24.00000000000000000, 110.0000000000000000, 30.00000000000000000 ) ) ;
#5912=DIRECTION ( 'NONE',  ( -1.000000000000000000, 0.000000000000000000, -0.000000000000000000 ) ) ;
#5918=LINE ( 'NONE', #2877, #10288 ) ;
#5921=EDGE_CURVE ( 'NONE', #7863, #13130, #19220, .T. ) ;
#5927=CARTESIAN_POINT ( 'NONE',  ( -41.00000000000000711, 53.00000000000000711, 6.999999999999999112 ) ) ;
#5933=VECTOR ( 'NONE', #13417, 1000.000000000000000 ) ;
#5935=EDGE_CURVE ( 'NONE', #9405, #12335, #13124, .T. ) ;
#5940=VECTOR ( 'NONE', #11369, 1000.000000000000000 ) ;
#5944=CARTESIAN_POINT ( 'NONE',  ( -40.00000000000000711, 113.0000000000000000, 0.5000000000000004441 ) ) ;
#5945=FACE_OUTER_BOUND ( 'NONE', #7066, .T. ) ;
#5946=VECTOR ( 'NONE', #4722, 1000.000000000000000 ) ;
#5956=CARTESIAN_POINT ( 'NONE',  ( -41.00000000000000711, 53.00000000000000711, 13.50000000000000000 ) ) ;
#5957=VERTEX_POINT ( 'NONE', #10383 ) ;
#5960=CARTESIAN_POINT ( 'NONE',  ( -40.00000000000000711, 110.0000000000000000, 30.00000000000000000 ) ) ;
#5970=AXIS2_PLACEMENT_3D ( 'NONE', #8633, #7267, #5706 ) ;
#5976=CARTESIAN_POINT ( 'NONE',  ( -25.00000000000000000, 110.0000000000000000, 8.000000000000000000 ) ) ;
#5981=EDGE_LOOP ( 'NONE', ( #8881, #8921, #9288, #14834 ) ) ;
#6000=PLANE ( 'NONE',  #13799 ) ;
#6002=DIRECTION ( 'NONE',  ( 0.000000000000000000, 0.000000000000000000, 1.000000000000000000 ) ) ;
#6003=VECTOR ( 'NONE', #16284, 1000.000000000000000 ) ;
#6005=CARTESIAN_POINT ( 'NONE',  ( -32.50000000000000000, 53.00000000000000711, 15.00000000000000000 ) ) ;
#6006=VECTOR ( 'NONE', #15782, 1000.000000000000000 ) ;
#6011=ORIENTED_EDGE ( 'NONE', *, *, #7360, .T. ) ;
#6014=CIRCLE ( 'NONE', #5084, 2.649999999999985700 ) ;
#6019=LINE ( 'NONE', #9044, #15044 ) ;
#6024=EDGE_CURVE ( 'NONE', #11249, #10297, #17749, .T. ) ;
#6027=FACE_OUTER_BOUND ( 'NONE', #4822, .T. ) ;
#6029=DIRECTION ( 'NONE',  ( 0.000000000000000000, 1.000000000000000000, 0.000000000000000000 ) ) ;
#6031=CARTESIAN_POINT ( 'NONE',  ( -41.00000000000000711, 53.00000000000000711, -32.00000000000000000 ) ) ;
#6060=DIRECTION ( 'NONE',  ( 1.000000000000000000, -0.000000000000000000, -0.000000000000000000 ) ) ;
#6064=ORIENTED_EDGE ( 'NONE', *, *, #8117, .T. ) ;
#6073=APPLICATION_CONTEXT ( 'automotive_design' ) ;
#6077=ORIENTED_EDGE ( 'NONE', *, *, #12009, .T. ) ;
#6086=CARTESIAN_POINT ( 'NONE',  ( -40.00000000000000711, 110.0000000000000000, 30.00000000000000000 ) ) ;
#6091=LINE ( 'NONE', #4627, #5049 ) ;
#6102=VECTOR ( 'NONE', #2621, 1000.000000000000000 ) ;
#6118=FACE_OUTER_BOUND ( 'NONE', #3223, .T. ) ;
#6124=AXIS2_PLACEMENT_3D ( 'NONE', #12697, #15560, #10940 ) ;
#6126=EDGE_CURVE ( 'NONE', #12927, #8090, #8384, .T. ) ;
#6139=VECTOR ( 'NONE', #18132, 1000.000000000000000 ) ;
#6141=LINE ( 'NONE', #7608, #8726 ) ;
#6143=AXIS2_PLACEMENT_3D ( 'NONE', #12388, #141, #7690 ) ;
#6145=DIRECTION ( 'NONE',  ( 1.000000000000000000, -0.000000000000000000, -0.000000000000000000 ) ) ;
#6149=EDGE_CURVE ( 'NONE', #12140, #17031, #11697, .T. ) ;
#6151=LINE ( 'NONE', #8089, #10826 ) ;
#6158=ORIENTED_EDGE ( 'NONE', *, *, #7349, .T. ) ;
#6166=ORIENTED_EDGE ( 'NONE', *, *, #15643, .T. ) ;
#6168=CARTESIAN_POINT ( 'NONE',  ( -40.00000000000000711, 110.0000000000000000, 13.50000000000000178 ) ) ;
#6186=( NAMED_UNIT ( * ) PLANE_ANGLE_UNIT ( ) SI_UNIT ( $, .RADIAN. ) );
#6193=VERTEX_POINT ( 'NONE', #14939 ) ;
#6196=ORIENTED_EDGE ( 'NONE', *, *, #4140, .F. ) ;
#6200=CARTESIAN_POINT ( 'NONE',  ( -40.00000000000000000, 53.00000000000000711, -50.00000000000000000 ) ) ;
#6214=ORIENTED_EDGE ( 'NONE', *, *, #3470, .T. ) ;
#6219=DIRECTION ( 'NONE',  ( -1.000000000000000000, 0.000000000000000000, -0.000000000000000000 ) ) ;
#6220=DIRECTION ( 'NONE',  ( 0.000000000000000000, 0.000000000000000000, -1.000000000000000000 ) ) ;
#6223=DIRECTION ( 'NONE',  ( 0.000000000000000000, -1.000000000000000000, 0.000000000000000000 ) ) ;
#6233=DIRECTION ( 'NONE',  ( 0.000000000000000000, 0.000000000000000000, 1.000000000000000000 ) ) ;
#6239=LINE ( 'NONE', #2900, #8396 ) ;
#6241=CARTESIAN_POINT ( 'NONE',  ( -41.00000000000000711, 110.0000000000000000, -11.50000000000000000 ) ) ;
#6242=PLANE ( 'NONE',  #9602 ) ;
#6244=DIRECTION ( 'NONE',  ( 1.000000000000000000, -0.000000000000000000, -0.000000000000000000 ) ) ;
#6245=ORIENTED_EDGE ( 'NONE', *, *, #12226, .T. ) ;
#6248=ADVANCED_FACE ( 'NONE', ( #1408 ), #19155, .T. ) ;
#6268=DIRECTION ( 'NONE',  ( 1.000000000000000000, -0.000000000000000000, -0.000000000000000000 ) ) ;
#6271=ORIENTED_EDGE ( 'NONE', *, *, #16937, .T. ) ;
#6273=ORIENTED_EDGE ( 'NONE', *, *, #18853, .F. ) ;
#6275=ORIENTED_EDGE ( 'NONE', *, *, #2439, .F. ) ;
#6291=ORIENTED_EDGE ( 'NONE', *, *, #7103, .F. ) ;
#6295=CARTESIAN_POINT ( 'NONE',  ( -24.00000000000000000, 53.00000000000000711, 30.00000000000000000 ) ) ;
#6299=CARTESIAN_POINT ( 'NONE',  ( -25.00000000000000000, 110.0000000000000000, 30.00000000000000000 ) ) ;
#6305=VECTOR ( 'NONE', #12433, 1000.000000000000000 ) ;
#6320=PLANE ( 'NONE',  #8178 ) ;
#6321=LINE ( 'NONE', #1805, #8157 ) ;
#6322=VECTOR ( 'NONE', #15847, 1000.000000000000000 ) ;
#6325=CARTESIAN_POINT ( 'NONE',  ( -24.00000000000000000, 53.00000000000000711, -38.50000000000000711 ) ) ;
#6335=CARTESIAN_POINT ( 'NONE',  ( -41.00000000000000711, 53.00000000000000711, 27.50000000000000000 ) ) ;
#6343=LINE ( 'NONE', #17026, #15614 ) ;
#6351=EDGE_LOOP ( 'NONE', ( #6696, #10283, #12733, #7946 ) ) ;
#6358=PLANE ( 'NONE',  #6124 ) ;
#6368=CARTESIAN_POINT ( 'NONE',  ( -25.00000000000000000, 110.0000000000000000, 14.50000000000000000 ) ) ;
#6372=EDGE_LOOP ( 'NONE', ( #6758, #3739, #17530, #12715 ) ) ;
#6377=ORIENTED_EDGE ( 'NONE', *, *, #2203, .T. ) ;
#6384=ORIENTED_EDGE ( 'NONE', *, *, #8459, .T. ) ;
#6392=DIRECTION ( 'NONE',  ( 0.000000000000000000, 0.000000000000000000, -1.000000000000000000 ) ) ;
#6397=DIRECTION ( 'NONE',  ( 0.000000000000000000, 1.000000000000000000, 0.000000000000000000 ) ) ;
#6411=CARTESIAN_POINT ( 'NONE',  ( -41.00000000000000711, 53.00000000000000711, 0.5000000000000004441 ) ) ;
#6414=CARTESIAN_POINT ( 'NONE',  ( -24.00000000000000000, 110.0000000000000000, 30.00000000000000000 ) ) ;
#6424=EDGE_CURVE ( 'NONE', #2590, #18664, #1996, .T. ) ;
#6437=DIRECTION ( 'NONE',  ( -0.000000000000000000, -0.000000000000000000, -1.000000000000000000 ) ) ;
#6439=VECTOR ( 'NONE', #3148, 1000.000000000000000 ) ;
#6442=CARTESIAN_POINT ( 'NONE',  ( -40.00000000000000000, 53.00000000000000711, 30.00000000000000000 ) ) ;
#6452=AXIS2_PLACEMENT_3D ( 'NONE', #2956, #5713, #13434 ) ;
#6456=ORIENTED_EDGE ( 'NONE', *, *, #16510, .T. ) ;
#6457=ORIENTED_EDGE ( 'NONE', *, *, #15060, .F. ) ;
#6463=CARTESIAN_POINT ( 'NONE',  ( -40.00000000000000711, 113.0000000000000000, 30.00000000000000000 ) ) ;
#6469=ORIENTED_EDGE ( 'NONE', *, *, #11513, .F. ) ;
#6480=VECTOR ( 'NONE', #8529, 1000.000000000000000 ) ;
#6485=ORIENTED_EDGE ( 'NONE', *, *, #5935, .T. ) ;
#6489=FACE_BOUND ( 'NONE', #15711, .T. ) ;
#6497=ORIENTED_EDGE ( 'NONE', *, *, #3754, .T. ) ;
#6508=CARTESIAN_POINT ( 'NONE',  ( -24.00000000000000000, 53.00000000000000711, -50.00000000000000000 ) ) ;
#6514=EDGE_CURVE ( 'NONE', #993, #17457, #14423, .T. ) ;
#6518=VERTEX_POINT ( 'NONE', #11280 ) ;
#6524=DIRECTION ( 'NONE',  ( 0.000000000000000000, -1.000000000000000000, 0.000000000000000000 ) ) ;
#6534=LINE ( 'NONE', #13778, #14142 ) ;
#6538=VECTOR ( 'NONE', #2210, 1000.000000000000000 ) ;
#6553=VERTEX_POINT ( 'NONE', #17365 ) ;
#6571=ADVANCED_FACE ( 'NONE', ( #11187 ), #12940, .T. ) ;
#6586=FACE_BOUND ( 'NONE', #16261, .T. ) ;
#6591=DIRECTION ( 'NONE',  ( 1.000000000000000000, -0.000000000000000000, -0.000000000000000000 ) ) ;
#6600=VECTOR ( 'NONE', #10132, 1000.000000000000000 ) ;
#6601=EDGE_CURVE ( 'NONE', #185, #7469, #17458, .T. ) ;
#6606=ORIENTED_EDGE ( 'NONE', *, *, #12234, .T. ) ;
#6607=AXIS2_PLACEMENT_3D ( 'NONE', #1696, #3167, #5912 ) ;
#6611=CARTESIAN_POINT ( 'NONE',  ( -25.00000000000000000, 113.0000000000000000, 30.00000000000000000 ) ) ;
#6624=VECTOR ( 'NONE', #532, 1000.000000000000000 ) ;
#6628=DIRECTION ( 'NONE',  ( 1.000000000000000000, -0.000000000000000000, -0.000000000000000000 ) ) ;
#6635=VECTOR ( 'NONE', #16829, 1000.000000000000000 ) ;
#6636=CARTESIAN_POINT ( 'NONE',  ( -41.00000000000000711, 110.0000000000000000, 21.00000000000000000 ) ) ;
#6639=EDGE_CURVE ( 'NONE', #19248, #1662, #17859, .T. ) ;
#6640=VERTEX_POINT ( 'NONE', #8833 ) ;
#6660=VERTEX_POINT ( 'NONE', #19133 ) ;
#6665=ORIENTED_EDGE ( 'NONE', *, *, #14433, .T. ) ;
#6667=ADVANCED_FACE ( 'NONE', ( #16385 ), #4139, .F. ) ;
#6673=VERTEX_POINT ( 'NONE', #1291 ) ;
#6678=ORIENTED_EDGE ( 'NONE', *, *, #15149, .T. ) ;
#6696=ORIENTED_EDGE ( 'NONE', *, *, #9412, .F. ) ;
#6697=DIRECTION ( 'NONE',  ( 1.156482317317871478E-16, -1.000000000000000000, 0.000000000000000000 ) ) ;
#6702=CARTESIAN_POINT ( 'NONE',  ( -25.00000000000000000, 53.00000000000000711, -44.00000000000000000 ) ) ;
#6704=EDGE_LOOP ( 'NONE', ( #19311, #1947, #12918, #12996 ) ) ;
#6714=LINE ( 'NONE', #5343, #5301 ) ;
#6717=DIRECTION ( 'NONE',  ( 1.000000000000000000, -0.000000000000000000, -0.000000000000000000 ) ) ;
#6721=ADVANCED_FACE ( 'NONE', ( #7560 ), #6000, .F. ) ;
#6733=VERTEX_POINT ( 'NONE', #14713 ) ;
#6734=CARTESIAN_POINT ( 'NONE',  ( -25.00000000000000711, 53.00000000000000711, -45.00000000000000000 ) ) ;
#6738=ADVANCED_FACE ( 'NONE', ( #5797 ), #11760, .T. ) ;
#6743=EDGE_CURVE ( 'NONE', #16834, #4224, #10286, .T. ) ;
#6747=( NAMED_UNIT ( * ) PLANE_ANGLE_UNIT ( ) SI_UNIT ( $, .RADIAN. ) );
#6748=VERTEX_POINT ( 'NONE', #13332 ) ;
#6751=ORIENTED_EDGE ( 'NONE', *, *, #14501, .F. ) ;
#6757=PLANE ( 'NONE',  #15338 ) ;
#6758=ORIENTED_EDGE ( 'NONE', *, *, #7372, .F. ) ;
#6760=FACE_OUTER_BOUND ( 'NONE', #10102, .T. ) ;
#6763=EDGE_CURVE ( 'NONE', #13282, #4488, #16485, .T. ) ;
#6764=CARTESIAN_POINT ( 'NONE',  ( -25.00000000000000711, 53.00000000000000711, -37.50000000000000711 ) ) ;
#6778=ORIENTED_EDGE ( 'NONE', *, *, #18605, .F. ) ;
#6785=DIRECTION ( 'NONE',  ( 0.000000000000000000, 1.000000000000000000, 0.000000000000000000 ) ) ;
#6794=DIRECTION ( 'NONE',  ( 1.000000000000000000, 0.000000000000000000, 0.000000000000000000 ) ) ;
#6795=STYLED_ITEM ( 'NONE', ( #2420 ), #11089 ) ;
#6797=CARTESIAN_POINT ( 'NONE',  ( -24.00000000000000711, 53.00000000000000711, 26.50000000000000000 ) ) ;
#6813=CARTESIAN_POINT ( 'NONE',  ( -41.00000000000000711, 110.0000000000000000, -31.00000000000000000 ) ) ;
#6816=ORIENTED_EDGE ( 'NONE', *, *, #4645, .T. ) ;
#6820=FACE_OUTER_BOUND ( 'NONE', #13893, .T. ) ;
#6823=VERTEX_POINT ( 'NONE', #1877 ) ;
#6824=CARTESIAN_POINT ( 'NONE',  ( -40.00000000000000000, 53.00000000000000711, 30.00000000000000000 ) ) ;
#6827=CARTESIAN_POINT ( 'NONE',  ( -24.00000000000000000, 53.00000000000000711, 30.00000000000000000 ) ) ;
#6828=AXIS2_PLACEMENT_3D ( 'NONE', #5649, #13185, #11611 ) ;
#6843=DIRECTION ( 'NONE',  ( 0.000000000000000000, 0.000000000000000000, -1.000000000000000000 ) ) ;
#6846=CARTESIAN_POINT ( 'NONE',  ( -41.00000000000000711, 110.0000000000000000, 8.000000000000000000 ) ) ;
#6856=AXIS2_PLACEMENT_3D ( 'NONE', #16878, #14124, #2070 ) ;
#6857=LINE ( 'NONE', #17349, #10813 ) ;
#6859=ORIENTED_EDGE ( 'NONE', *, *, #15468, .F. ) ;
#6862=CARTESIAN_POINT ( 'NONE',  ( -24.00000000000000000, 110.0000000000000000, -25.49999999999999645 ) ) ;
#6865=EDGE_CURVE ( 'NONE', #5230, #17811, #13535, .T. ) ;
#6875=LINE ( 'NONE', #11465, #11541 ) ;
#6876=ORIENTED_EDGE ( 'NONE', *, *, #3646, .T. ) ;
#6883=FACE_BOUND ( 'NONE', #3127, .T. ) ;
#6885=DIRECTION ( 'NONE',  ( 0.000000000000000000, 0.000000000000000000, -1.000000000000000000 ) ) ;
#6890=EDGE_LOOP ( 'NONE', ( #8389, #12934, #16895, #17374 ) ) ;
#6920=ORIENTED_EDGE ( 'NONE', *, *, #659, .T. ) ;
#6928=EDGE_CURVE ( 'NONE', #2358, #7475, #12059, .T. ) ;
#6931=ORIENTED_EDGE ( 'NONE', *, *, #2994, .F. ) ;
#6934=AXIS2_PLACEMENT_3D ( 'NONE', #18896, #11330, #17233 ) ;
#6935=ORIENTED_EDGE ( 'NONE', *, *, #13803, .T. ) ;
#6936=VERTEX_POINT ( 'NONE', #6200 ) ;
#6943=DIRECTION ( 'NONE',  ( 0.000000000000000000, 1.000000000000000000, 0.000000000000000000 ) ) ;
#6945=LINE ( 'NONE', #16058, #4749 ) ;
#6947=DIRECTION ( 'NONE',  ( 0.000000000000000000, -1.000000000000000000, -0.000000000000000000 ) ) ;
#6957=ORIENTED_EDGE ( 'NONE', *, *, #3381, .T. ) ;
#6964=EDGE_CURVE ( 'NONE', #3115, #11249, #2910, .T. ) ;
#6966=EDGE_LOOP ( 'NONE', ( #9123, #2182, #2046, #13132 ) ) ;
#6968=EDGE_CURVE ( 'NONE', #14875, #16369, #19287, .T. ) ;
#6969=DIRECTION ( 'NONE',  ( 0.000000000000000000, 0.000000000000000000, -1.000000000000000000 ) ) ;
#6994=FACE_OUTER_BOUND ( 'NONE', #10550, .T. ) ;
#6997=EDGE_CURVE ( 'NONE', #9604, #14297, #16439, .T. ) ;
#7007=VECTOR ( 'NONE', #11191, 1000.000000000000000 ) ;
#7023=ORIENTED_EDGE ( 'NONE', *, *, #10575, .F. ) ;
#7028=ORIENTED_EDGE ( 'NONE', *, *, #15149, .F. ) ;
#7032=AXIS2_PLACEMENT_3D ( 'NONE', #6295, #4830, #16781 ) ;
#7039=CARTESIAN_POINT ( 'NONE',  ( -24.00000000000000000, 110.0000000000000000, 6.999999999999999112 ) ) ;
#7040=ORIENTED_EDGE ( 'NONE', *, *, #18302, .F. ) ;
#7043=CARTESIAN_POINT ( 'NONE',  ( -32.50000000000000000, 52.00000000000000711, -35.00000000000000000 ) ) ;
#7050=VERTEX_POINT ( 'NONE', #16346 ) ;
#7065=LINE ( 'NONE', #10090, #16907 ) ;
#7066=EDGE_LOOP ( 'NONE', ( #2807, #5136, #5876, #16194 ) ) ;
#7074=DIRECTION ( 'NONE',  ( -1.156482317317871725E-16, 1.000000000000000000, 0.000000000000000000 ) ) ;
#7075=DIRECTION ( 'NONE',  ( 0.000000000000000000, 0.000000000000000000, 1.000000000000000000 ) ) ;
#7078=CARTESIAN_POINT ( 'NONE',  ( -41.00000000000000711, 53.00000000000000711, 8.000000000000000000 ) ) ;
#7086=ORIENTED_EDGE ( 'NONE', *, *, #16547, .F. ) ;
#7087=CARTESIAN_POINT ( 'NONE',  ( -40.00000000000000000, 53.00000000000000711, 30.00000000000000000 ) ) ;
#7093=CARTESIAN_POINT ( 'NONE',  ( -41.00000000000000711, 53.00000000000000711, 6.999999999999999112 ) ) ;
#7103=EDGE_CURVE ( 'NONE', #18913, #1793, #12966, .T. ) ;
#7115=FACE_OUTER_BOUND ( 'NONE', #9891, .T. ) ;
#7119=EDGE_CURVE ( 'NONE', #13602, #13902, #9247, .T. ) ;
#7127=ORIENTED_EDGE ( 'NONE', *, *, #14798, .T. ) ;
#7135=VERTEX_POINT ( 'NONE', #3175 ) ;
#7137=VERTEX_POINT ( 'NONE', #7685 ) ;
#7148=VERTEX_POINT ( 'NONE', #18082 ) ;
#7150=VECTOR ( 'NONE', #16026, 1000.000000000000000 ) ;
#7152=ORIENTED_EDGE ( 'NONE', *, *, #9532, .T. ) ;
#7159=ORIENTED_EDGE ( 'NONE', *, *, #7605, .F. ) ;
#7164=VECTOR ( 'NONE', #353, 1000.000000000000000 ) ;
#7175=VECTOR ( 'NONE', #9529, 1000.000000000000000 ) ;
#7177=VECTOR ( 'NONE', #17729, 1000.000000000000000 ) ;
#7181=ORIENTED_EDGE ( 'NONE', *, *, #18854, .F. ) ;
#7182=CARTESIAN_POINT ( 'NONE',  ( -41.00000000000000711, 53.00000000000000711, 26.50000000000000000 ) ) ;
#7190=LINE ( 'NONE', #17391, #7150 ) ;
#7194=DIRECTION ( 'NONE',  ( 0.000000000000000000, -1.000000000000000000, -0.000000000000000000 ) ) ;
#7197=ADVANCED_FACE ( 'NONE', ( #6027 ), #7589, .F. ) ;
#7198=EDGE_CURVE ( 'NONE', #209, #17838, #19353, .T. ) ;
#7201=VECTOR ( 'NONE', #1751, 1000.000000000000000 ) ;
#7214=VECTOR ( 'NONE', #13556, 1000.000000000000000 ) ;
#7217=PLANE ( 'NONE',  #967 ) ;
#7219=VECTOR ( 'NONE', #759, 1000.000000000000000 ) ;
#7221=ORIENTED_EDGE ( 'NONE', *, *, #15617, .T. ) ;
#7227=EDGE_LOOP ( 'NONE', ( #11438, #5382, #10988, #12802 ) ) ;
#7233=ORIENTED_EDGE ( 'NONE', *, *, #2492, .T. ) ;
#7234=VERTEX_POINT ( 'NONE', #16408 ) ;
#7241=LINE ( 'NONE', #11353, #3748 ) ;
#7250=ORIENTED_EDGE ( 'NONE', *, *, #18974, .F. ) ;
#7253=ADVANCED_FACE ( 'NONE', ( #14944 ), #6320, .F. ) ;
#7267=DIRECTION ( 'NONE',  ( 0.000000000000000000, 0.000000000000000000, -1.000000000000000000 ) ) ;
#7283=CARTESIAN_POINT ( 'NONE',  ( -25.00000000000000000, 110.0000000000000000, 30.00000000000000000 ) ) ;
#7284=ORIENTED_EDGE ( 'NONE', *, *, #12644, .F. ) ;
#7306=DIRECTION ( 'NONE',  ( 1.000000000000000000, -0.000000000000000000, -0.000000000000000000 ) ) ;
#7316=ORIENTED_EDGE ( 'NONE', *, *, #14178, .T. ) ;
#7318=EDGE_CURVE ( 'NONE', #12423, #4121, #15526, .T. ) ;
#7328=EDGE_LOOP ( 'NONE', ( #5115, #5854, #6457, #3533 ) ) ;
#7329=ORIENTED_EDGE ( 'NONE', *, *, #18148, .T. ) ;
#7330=CARTESIAN_POINT ( 'NONE',  ( -41.00000000000000711, 110.0000000000000000, 0.5000000000000004441 ) ) ;
#7331=VERTEX_POINT ( 'NONE', #18381 ) ;
#7333=VERTEX_POINT ( 'NONE', #11005 ) ;
#7335=CARTESIAN_POINT ( 'NONE',  ( -40.00000000000000711, 113.0000000000000000, 30.00000000000000000 ) ) ;
#7337=DIRECTION ( 'NONE',  ( 0.000000000000000000, 0.000000000000000000, -1.000000000000000000 ) ) ;
#7340=VERTEX_POINT ( 'NONE', #18754 ) ;
#7341=ORIENTED_EDGE ( 'NONE', *, *, #4508, .F. ) ;
#7344=DIRECTION ( 'NONE',  ( -1.000000000000000000, 0.000000000000000000, -0.000000000000000000 ) ) ;
#7345=EDGE_LOOP ( 'NONE', ( #19264, #12178, #6859, #14515 ) ) ;
#7346=AXIS2_PLACEMENT_3D ( 'NONE', #3771, #2112, #3385 ) ;
#7349=EDGE_CURVE ( 'NONE', #16683, #12144, #11099, .T. ) ;
#7353=EDGE_CURVE ( 'NONE', #6748, #7898, #5142, .T. ) ;
#7359=CARTESIAN_POINT ( 'NONE',  ( -41.00000000000000711, 110.0000000000000000, -44.00000000000000000 ) ) ;
#7360=EDGE_CURVE ( 'NONE', #8784, #7135, #15434, .T. ) ;
#7363=FACE_OUTER_BOUND ( 'NONE', #1863, .T. ) ;
#7366=CARTESIAN_POINT ( 'NONE',  ( -40.00000000000000711, 113.0000000000000000, -31.00000000000000000 ) ) ;
#7372=EDGE_CURVE ( 'NONE', #2358, #3528, #9724, .T. ) ;
#7381=VERTEX_POINT ( 'NONE', #11282 ) ;
#7385=CARTESIAN_POINT ( 'NONE',  ( -41.00000000000000711, 53.00000000000000711, -6.000000000000001776 ) ) ;
#7387=DIRECTION ( 'NONE',  ( 0.000000000000000000, 1.000000000000000000, 0.000000000000000000 ) ) ;
#7390=VECTOR ( 'NONE', #534, 1000.000000000000000 ) ;
#7391=AXIS2_PLACEMENT_3D ( 'NONE', #12584, #13957, #18578 ) ;
#7393=DIRECTION ( 'NONE',  ( 1.000000000000000000, -0.000000000000000000, -0.000000000000000000 ) ) ;
#7402=VECTOR ( 'NONE', #9618, 1000.000000000000000 ) ;
#7411=CARTESIAN_POINT ( 'NONE',  ( -40.00000000000000711, 110.0000000000000000, -24.49999999999999645 ) ) ;
#7417=ORIENTED_EDGE ( 'NONE', *, *, #9608, .T. ) ;
#7422=ORIENTED_EDGE ( 'NONE', *, *, #18079, .T. ) ;
#7432=ORIENTED_EDGE ( 'NONE', *, *, #132, .T. ) ;
#7440=EDGE_LOOP ( 'NONE', ( #16773, #18040, #8571, #15874 ) ) ;
#7449=DIRECTION ( 'NONE',  ( 1.000000000000000000, -0.000000000000000000, -0.000000000000000000 ) ) ;
#7450=DIRECTION ( 'NONE',  ( 0.000000000000000000, 0.000000000000000000, 1.000000000000000000 ) ) ;
#7451=ORIENTED_EDGE ( 'NONE', *, *, #7860, .T. ) ;
#7469=VERTEX_POINT ( 'NONE', #12759 ) ;
#7474=CARTESIAN_POINT ( 'NONE',  ( -40.00000000000000711, 53.00000000000000711, -5.000000000000000888 ) ) ;
#7475=VERTEX_POINT ( 'NONE', #3372 ) ;
#7478=CARTESIAN_POINT ( 'NONE',  ( -41.00000000000000711, 53.00000000000000711, -30.99999999999999645 ) ) ;
#7484=VECTOR ( 'NONE', #5482, 1000.000000000000000 ) ;
#7485=EDGE_CURVE ( 'NONE', #16704, #19125, #525, .T. ) ;
#7486=CARTESIAN_POINT ( 'NONE',  ( -32.50000000000000000, 53.00000000000000711, 12.35000000000001386 ) ) ;
#7488=LINE ( 'NONE', #9250, #11133 ) ;
#7502=VECTOR ( 'NONE', #6697, 1000.000000000000000 ) ;
#7505=EDGE_CURVE ( 'NONE', #1057, #6748, #5506, .T. ) ;
#7512=AXIS2_PLACEMENT_3D ( 'NONE', #17586, #5626, #1317 ) ;
#7516=ORIENTED_EDGE ( 'NONE', *, *, #14558, .T. ) ;
#7521=ORIENTED_EDGE ( 'NONE', *, *, #8879, .F. ) ;
#7533=ORIENTED_EDGE ( 'NONE', *, *, #16694, .F. ) ;
#7546=AXIS2_PLACEMENT_3D ( 'NONE', #14470, #755, #2322 ) ;
#7557=DIRECTION ( 'NONE',  ( 1.000000000000000000, -0.000000000000000000, -0.000000000000000000 ) ) ;
#7560=FACE_OUTER_BOUND ( 'NONE', #16967, .T. ) ;
#7563=CIRCLE ( 'NONE', #47, 2.649999999999999467 ) ;
#7589=PLANE ( 'NONE',  #14408 ) ;
#7595=ORIENTED_EDGE ( 'NONE', *, *, #4746, .F. ) ;
#7602=EDGE_CURVE ( 'NONE', #7381, #10051, #15899, .T. ) ;
#7605=EDGE_CURVE ( 'NONE', #7955, #8804, #17460, .T. ) ;
#7606=CARTESIAN_POINT ( 'NONE',  ( -24.00000000000000711, 53.00000000000000711, -38.50000000000000711 ) ) ;
#7608=CARTESIAN_POINT ( 'NONE',  ( -32.50000000000000000, 53.00000000000000711, -32.35000000000000853 ) ) ;
#7613=PLANE ( 'NONE',  #13500 ) ;
#7620=ORIENTED_EDGE ( 'NONE', *, *, #18620, .T. ) ;
#7623=ORIENTED_EDGE ( 'NONE', *, *, #11929, .T. ) ;
#7631=VERTEX_POINT ( 'NONE', #10094 ) ;
#7632=ORIENTED_EDGE ( 'NONE', *, *, #15381, .F. ) ;
#7634=CARTESIAN_POINT ( 'NONE',  ( -25.00000000000000711, 53.00000000000000711, 14.50000000000000000 ) ) ;
#7640=CARTESIAN_POINT ( 'NONE',  ( -41.00000000000000711, 53.00000000000000711, -44.00000000000000000 ) ) ;
#7646=DIRECTION ( 'NONE',  ( 1.000000000000000000, 0.000000000000000000, 0.000000000000000000 ) ) ;
#7659=EDGE_LOOP ( 'NONE', ( #13710, #4811, #8605, #1356 ) ) ;
#7660=CARTESIAN_POINT ( 'NONE',  ( -41.00000000000000711, 53.00000000000000711, -5.000000000000000888 ) ) ;
#7665=DIRECTION ( 'NONE',  ( -0.000000000000000000, -0.000000000000000000, -1.000000000000000000 ) ) ;
#7671=CARTESIAN_POINT ( 'NONE',  ( -41.00000000000000711, 110.0000000000000000, -45.00000000000000000 ) ) ;
#7681=DIRECTION ( 'NONE',  ( -0.000000000000000000, -0.000000000000000000, -1.000000000000000000 ) ) ;
#7685=CARTESIAN_POINT ( 'NONE',  ( -41.00000000000000711, 110.0000000000000000, 1.500000000000001332 ) ) ;
#7690=DIRECTION ( 'NONE',  ( 0.000000000000000000, 0.000000000000000000, -1.000000000000000000 ) ) ;
#7692=VECTOR ( 'NONE', #16531, 1000.000000000000000 ) ;
#7694=ORIENTED_EDGE ( 'NONE', *, *, #12293, .F. ) ;
#7705=LINE ( 'NONE', #14067, #7164 ) ;
#7709=CARTESIAN_POINT ( 'NONE',  ( -41.00000000000000711, 53.00000000000000711, -30.99999999999999645 ) ) ;
#7710=LINE ( 'NONE', #6241, #19147 ) ;
#7711=DIRECTION ( 'NONE',  ( -1.000000000000000000, 0.000000000000000000, -0.000000000000000000 ) ) ;
#7714=EDGE_CURVE ( 'NONE', #6553, #11839, #13236, .T. ) ;
#7715=EDGE_CURVE ( 'NONE', #15519, #2028, #17760, .T. ) ;
#7719=EDGE_CURVE ( 'NONE', #18999, #5693, #1389, .T. ) ;
#7723=VECTOR ( 'NONE', #8011, 1000.000000000000000 ) ;
#7743=CARTESIAN_POINT ( 'NONE',  ( -41.00000000000000711, 110.0000000000000000, 27.50000000000000000 ) ) ;
#7749=ORIENTED_EDGE ( 'NONE', *, *, #7972, .T. ) ;
#7755=LINE ( 'NONE', #2843, #928 ) ;
#7761=EDGE_LOOP ( 'NONE', ( #14913, #11961, #11235, #14606 ) ) ;
#7764=PLANE ( 'NONE',  #7032 ) ;
#7765=LINE ( 'NONE', #10394, #10670 ) ;
#7774=CARTESIAN_POINT ( 'NONE',  ( -41.00000000000000711, 110.0000000000000000, -38.50000000000000711 ) ) ;
#7775=ORIENTED_EDGE ( 'NONE', *, *, #15915, .T. ) ;
#7777=ADVANCED_FACE ( 'NONE', ( #7363 ), #15013, .F. ) ;
#7784=LINE ( 'NONE', #13752, #3301 ) ;
#7786=EDGE_CURVE ( 'NONE', #17050, #1646, #1589, .T. ) ;
#7808=PLANE ( 'NONE',  #5226 ) ;
#7812=LINE ( 'NONE', #6442, #18966 ) ;
#7813=ORIENTED_EDGE ( 'NONE', *, *, #3571, .F. ) ;
#7817=AXIS2_PLACEMENT_3D ( 'NONE', #7478, #17881, #35 ) ;
#7822=DIRECTION ( 'NONE',  ( -1.000000000000000000, 0.000000000000000000, -0.000000000000000000 ) ) ;
#7824=AXIS2_PLACEMENT_3D ( 'NONE', #12301, #18296, #17675 ) ;
#7831=CARTESIAN_POINT ( 'NONE',  ( -41.00000000000000711, 110.0000000000000000, -19.00000000000000000 ) ) ;
#7832=EDGE_CURVE ( 'NONE', #1050, #15591, #7765, .T. ) ;
#7834=EDGE_LOOP ( 'NONE', ( #18789, #6273, #17012, #4905 ) ) ;
#7838=EDGE_CURVE ( 'NONE', #11652, #7898, #9129, .T. ) ;
#7842=VECTOR ( 'NONE', #13007, 1000.000000000000000 ) ;
#7845=ORIENTED_EDGE ( 'NONE', *, *, #3754, .F. ) ;
#7850=ORIENTED_EDGE ( 'NONE', *, *, #3682, .F. ) ;
#7854=CARTESIAN_POINT ( 'NONE',  ( -25.00000000000000711, 53.00000000000000711, -18.00000000000000000 ) ) ;
#7860=EDGE_CURVE ( 'NONE', #17638, #11652, #14, .T. ) ;
#7863=VERTEX_POINT ( 'NONE', #9223 ) ;
#7887=ORIENTED_EDGE ( 'NONE', *, *, #8436, .T. ) ;
#7891=CARTESIAN_POINT ( 'NONE',  ( -41.00000000000000711, 53.00000000000000711, -5.000000000000000888 ) ) ;
#7892=CARTESIAN_POINT ( 'NONE',  ( -41.00000000000000711, 53.00000000000000711, -37.50000000000000711 ) ) ;
#7893=VECTOR ( 'NONE', #8121, 1000.000000000000000 ) ;
#7898=VERTEX_POINT ( 'NONE', #10289 ) ;
#7904=DIRECTION ( 'NONE',  ( 0.000000000000000000, -1.000000000000000000, 0.000000000000000000 ) ) ;
#7931=ADVANCED_FACE ( 'NONE', ( #2854 ), #8835, .T. ) ;
#7933=DIRECTION ( 'NONE',  ( 1.000000000000000000, -0.000000000000000000, -0.000000000000000000 ) ) ;
#7937=EDGE_CURVE ( 'NONE', #19283, #13814, #9513, .T. ) ;
#7940=EDGE_CURVE ( 'NONE', #9239, #14297, #1882, .T. ) ;
#7944=VERTEX_POINT ( 'NONE', #3445 ) ;
#7946=ORIENTED_EDGE ( 'NONE', *, *, #4704, .F. ) ;
#7955=VERTEX_POINT ( 'NONE', #13898 ) ;
#7967=CARTESIAN_POINT ( 'NONE',  ( -32.50000000000000000, 53.00000000000000711, 15.00000000000000000 ) ) ;
#7971=DIRECTION ( 'NONE',  ( 0.000000000000000000, 0.000000000000000000, -1.000000000000000000 ) ) ;
#7972=EDGE_CURVE ( 'NONE', #2146, #12847, #3326, .T. ) ;
#7978=DIRECTION ( 'NONE',  ( 0.000000000000000000, 0.000000000000000000, -1.000000000000000000 ) ) ;
#7982=CARTESIAN_POINT ( 'NONE',  ( -40.00000000000000711, 113.0000000000000000, -37.50000000000000711 ) ) ;
#7985=DIRECTION ( 'NONE',  ( 1.000000000000000000, -0.000000000000000000, -0.000000000000000000 ) ) ;
#7986=VECTOR ( 'NONE', #1212, 1000.000000000000000 ) ;
#7999=LINE ( 'NONE', #13965, #18240 ) ;
#8007=VECTOR ( 'NONE', #10372, 1000.000000000000000 ) ;
#8008=LINE ( 'NONE', #13976, #6635 ) ;
#8011=DIRECTION ( 'NONE',  ( 0.000000000000000000, 1.000000000000000000, 0.000000000000000000 ) ) ;
#8013=DIRECTION ( 'NONE',  ( 0.000000000000000000, 0.000000000000000000, -1.000000000000000000 ) ) ;
#8015=VERTEX_POINT ( 'NONE', #3608 ) ;
#8038=VECTOR ( 'NONE', #8478, 1000.000000000000000 ) ;
#8040=EDGE_LOOP ( 'NONE', ( #17449, #18055, #1995, #3806 ) ) ;
#8044=VERTEX_POINT ( 'NONE', #1756 ) ;
#8056=CARTESIAN_POINT ( 'NONE',  ( -41.00000000000000711, 53.00000000000000711, -32.00000000000000000 ) ) ;
#8061=ADVANCED_FACE ( 'NONE', ( #17323 ), #12709, .F. ) ;
#8062=DIRECTION ( 'NONE',  ( 1.000000000000000000, -0.000000000000000000, -0.000000000000000000 ) ) ;
#8066=FACE_OUTER_BOUND ( 'NONE', #14979, .T. ) ;
#8077=EDGE_LOOP ( 'NONE', ( #766, #13197, #11001, #14486 ) ) ;
#8082=CARTESIAN_POINT ( 'NONE',  ( -41.00000000000000711, 53.00000000000000711, -6.000000000000001776 ) ) ;
#8085=ADVANCED_FACE ( 'NONE', ( #944 ), #8494, .F. ) ;
#8086=CARTESIAN_POINT ( 'NONE',  ( -41.00000000000000711, 113.0000000000000000, 30.00000000000000000 ) ) ;
#8088=FACE_OUTER_BOUND ( 'NONE', #7328, .T. ) ;
#8089=CARTESIAN_POINT ( 'NONE',  ( -40.00000000000000711, 113.0000000000000000, -38.50000000000000711 ) ) ;
#8090=VERTEX_POINT ( 'NONE', #19079 ) ;
#8106=LINE ( 'NONE', #2306, #1445 ) ;
#8112=LINE ( 'NONE', #18700, #18022 ) ;
#8117=EDGE_CURVE ( 'NONE', #7050, #8090, #1042, .T. ) ;
#8121=DIRECTION ( 'NONE',  ( 1.000000000000000000, -0.000000000000000000, -0.000000000000000000 ) ) ;
#8130=ORIENTED_EDGE ( 'NONE', *, *, #656, .F. ) ;
#8134=ORIENTED_EDGE ( 'NONE', *, *, #12757, .T. ) ;
#8142=ORIENTED_EDGE ( 'NONE', *, *, #15071, .T. ) ;
#8153=CARTESIAN_POINT ( 'NONE',  ( -25.00000000000000000, 53.00000000000000711, 30.00000000000000000 ) ) ;
#8155=CARTESIAN_POINT ( 'NONE',  ( -40.00000000000000711, 113.0000000000000000, -24.49999999999999289 ) ) ;
#8157=VECTOR ( 'NONE', #13858, 1000.000000000000000 ) ;
#8168=CARTESIAN_POINT ( 'NONE',  ( -41.00000000000000711, 53.00000000000000711, -38.50000000000000711 ) ) ;
#8171=LINE ( 'NONE', #6508, #5615 ) ;
#8174=EDGE_CURVE ( 'NONE', #1049, #9, #7563, .T. ) ;
#8176=CARTESIAN_POINT ( 'NONE',  ( -41.00000000000000711, 53.00000000000000711, 27.50000000000000000 ) ) ;
#8178=AXIS2_PLACEMENT_3D ( 'NONE', #236, #6220, #8856 ) ;
#8184=ADVANCED_FACE ( 'NONE', ( #14768 ), #7613, .F. ) ;
#8211=DIRECTION ( 'NONE',  ( 0.000000000000000000, -1.000000000000000000, 0.000000000000000000 ) ) ;
#8212=EDGE_CURVE ( 'NONE', #12337, #14902, #13577, .T. ) ;
#8214=DIRECTION ( 'NONE',  ( 0.000000000000000000, 0.000000000000000000, -1.000000000000000000 ) ) ;
#8219=ORIENTED_EDGE ( 'NONE', *, *, #14433, .F. ) ;
#8223=CARTESIAN_POINT ( 'NONE',  ( -40.00000000000000711, 113.0000000000000000, -12.49999999999999645 ) ) ;
#8227=LINE ( 'NONE', #18331, #6305 ) ;
#8228=DIRECTION ( 'NONE',  ( -0.000000000000000000, -0.000000000000000000, -1.000000000000000000 ) ) ;
#8234=ORIENTED_EDGE ( 'NONE', *, *, #8212, .F. ) ;
#8241=ORIENTED_EDGE ( 'NONE', *, *, #8785, .F. ) ;
#8245=CARTESIAN_POINT ( 'NONE',  ( -40.00000000000000000, 53.00000000000000711, 30.00000000000000000 ) ) ;
#8251=DIRECTION ( 'NONE',  ( -1.000000000000000000, 0.000000000000000000, -0.000000000000000000 ) ) ;
#8259=DIRECTION ( 'NONE',  ( -1.000000000000000000, 0.000000000000000000, -0.000000000000000000 ) ) ;
#8262=DIRECTION ( 'NONE',  ( 0.000000000000000000, -1.000000000000000000, 0.000000000000000000 ) ) ;
#8265=DIRECTION ( 'NONE',  ( 1.000000000000000000, 0.000000000000000000, 0.000000000000000000 ) ) ;
#8268=CARTESIAN_POINT ( 'NONE',  ( -25.00000000000000000, 53.00000000000000711, 30.00000000000000000 ) ) ;
#8270=FACE_BOUND ( 'NONE', #1274, .T. ) ;
#8275=ORIENTED_EDGE ( 'NONE', *, *, #8117, .F. ) ;
#8302=DIRECTION ( 'NONE',  ( -1.156482317317871478E-16, 1.000000000000000000, 0.000000000000000000 ) ) ;
#8303=VECTOR ( 'NONE', #17281, 1000.000000000000000 ) ;
#8304=CARTESIAN_POINT ( 'NONE',  ( -41.00000000000000711, 110.0000000000000000, -11.50000000000000000 ) ) ;
#8306=CARTESIAN_POINT ( 'NONE',  ( -32.50000000000000000, 52.00000000000000711, 15.00000000000000000 ) ) ;
#8307=ADVANCED_FACE ( 'NONE', ( #5945 ), #11916, .F. ) ;
#8320=ORIENTED_EDGE ( 'NONE', *, *, #4037, .F. ) ;
#8342=ORIENTED_EDGE ( 'NONE', *, *, #8533, .F. ) ;
#8361=PLANE ( 'NONE',  #3888 ) ;
#8363=CARTESIAN_POINT ( 'NONE',  ( -41.00000000000000711, 110.0000000000000000, 27.50000000000000000 ) ) ;
#8366=VERTEX_POINT ( 'NONE', #5069 ) ;
#8372=DIRECTION ( 'NONE',  ( 0.000000000000000000, 0.000000000000000000, 1.000000000000000000 ) ) ;
#8384=LINE ( 'NONE', #14356, #4053 ) ;
#8389=ORIENTED_EDGE ( 'NONE', *, *, #16510, .F. ) ;
#8394=EDGE_CURVE ( 'NONE', #2269, #12927, #6534, .T. ) ;
#8396=VECTOR ( 'NONE', #10535, 1000.000000000000000 ) ;
#8420=DIRECTION ( 'NONE',  ( 0.000000000000000000, 0.000000000000000000, -1.000000000000000000 ) ) ;
#8421=CARTESIAN_POINT ( 'NONE',  ( -32.50000000000000000, 53.00000000000000711, -37.64999999999999858 ) ) ;
#8422=VECTOR ( 'NONE', #14278, 1000.000000000000000 ) ;
#8435=EDGE_CURVE ( 'NONE', #9439, #3017, #2018, .T. ) ;
#8436=EDGE_CURVE ( 'NONE', #5657, #16384, #8008, .T. ) ;
#8442=DIRECTION ( 'NONE',  ( 0.000000000000000000, 0.000000000000000000, -1.000000000000000000 ) ) ;
#8445=CARTESIAN_POINT ( 'NONE',  ( -40.00000000000000000, 52.00000000000000711, 30.00000000000000000 ) ) ;
#8451=VECTOR ( 'NONE', #432, 1000.000000000000000 ) ;
#8454=FACE_OUTER_BOUND ( 'NONE', #2407, .T. ) ;
#8457=LINE ( 'NONE', #7671, #14594 ) ;
#8459=EDGE_CURVE ( 'NONE', #16384, #14710, #7710, .T. ) ;
#8475=VECTOR ( 'NONE', #4426, 1000.000000000000000 ) ;
#8476=DIRECTION ( 'NONE',  ( 0.000000000000000000, 0.000000000000000000, 1.000000000000000000 ) ) ;
#8478=DIRECTION ( 'NONE',  ( 0.000000000000000000, -1.000000000000000000, 0.000000000000000000 ) ) ;
#8484=CARTESIAN_POINT ( 'NONE',  ( -25.00000000000000000, 53.00000000000000711, -5.000000000000004441 ) ) ;
#8487=ORIENTED_EDGE ( 'NONE', *, *, #625, .T. ) ;
#8494=PLANE ( 'NONE',  #6934 ) ;
#8495=DIRECTION ( 'NONE',  ( 1.000000000000000000, -0.000000000000000000, -0.000000000000000000 ) ) ;
#8500=ORIENTED_EDGE ( 'NONE', *, *, #9457, .T. ) ;
#8523=CARTESIAN_POINT ( 'NONE',  ( -41.00000000000000711, 53.00000000000000711, 13.50000000000000000 ) ) ;
#8525=ORIENTED_EDGE ( 'NONE', *, *, #2677, .F. ) ;
#8529=DIRECTION ( 'NONE',  ( 1.000000000000000000, -0.000000000000000000, -0.000000000000000000 ) ) ;
#8533=EDGE_CURVE ( 'NONE', #10285, #1200, #10632, .T. ) ;
#8535=EDGE_LOOP ( 'NONE', ( #15089, #10470, #19378, #14176 ) ) ;
#8537=CARTESIAN_POINT ( 'NONE',  ( -41.00000000000000711, 53.00000000000000711, 1.500000000000001332 ) ) ;
#8548=CARTESIAN_POINT ( 'NONE',  ( -41.00000000000000711, 53.00000000000000711, 21.00000000000000000 ) ) ;
#8551=DIRECTION ( 'NONE',  ( 1.000000000000000000, -0.000000000000000000, -0.000000000000000000 ) ) ;
#8560=LINE ( 'NONE', #12963, #17060 ) ;
#8562=FACE_OUTER_BOUND ( 'NONE', #8040, .T. ) ;
#8571=ORIENTED_EDGE ( 'NONE', *, *, #1582, .F. ) ;
#8602=DIRECTION ( 'NONE',  ( 0.000000000000000000, -1.000000000000000000, -0.000000000000000000 ) ) ;
#8603=ORIENTED_EDGE ( 'NONE', *, *, #2569, .F. ) ;
#8604=CARTESIAN_POINT ( 'NONE',  ( -41.00000000000000711, 53.00000000000000711, -32.00000000000000000 ) ) ;
#8605=ORIENTED_EDGE ( 'NONE', *, *, #4457, .F. ) ;
#8607=ORIENTED_EDGE ( 'NONE', *, *, #18100, .T. ) ;
#8610=DIRECTION ( 'NONE',  ( -0.000000000000000000, 1.000000000000000000, -0.000000000000000000 ) ) ;
#8619=ORIENTED_EDGE ( 'NONE', *, *, #14769, .F. ) ;
#8621=CARTESIAN_POINT ( 'NONE',  ( -41.00000000000000711, 110.0000000000000000, 20.00000000000000000 ) ) ;
#8624=DIRECTION ( 'NONE',  ( -0.000000000000000000, -0.000000000000000000, -1.000000000000000000 ) ) ;
#8625=ORIENTED_EDGE ( 'NONE', *, *, #9608, .F. ) ;
#8631=CARTESIAN_POINT ( 'NONE',  ( -25.00000000000000000, 53.00000000000000711, 30.00000000000000000 ) ) ;
#8633=CARTESIAN_POINT ( 'NONE',  ( -41.00000000000000711, 53.00000000000000711, 13.50000000000000000 ) ) ;
#8637=ADVANCED_FACE ( 'NONE', ( #5802 ), #2754, .T. ) ;
#8640=FACE_BOUND ( 'NONE', #5573, .T. ) ;
#8645=AXIS2_PLACEMENT_3D ( 'NONE', #15415, #115, #16785 ) ;
#8652=EDGE_CURVE ( 'NONE', #12114, #3704, #14764, .T. ) ;
#8666=ORIENTED_EDGE ( 'NONE', *, *, #11548, .T. ) ;
#8675=LINE ( 'NONE', #14366, #6322 ) ;
#8683=ORIENTED_EDGE ( 'NONE', *, *, #15071, .F. ) ;
#8686=ORIENTED_EDGE ( 'NONE', *, *, #2698, .F. ) ;
#8696=ORIENTED_EDGE ( 'NONE', *, *, #280, .T. ) ;
#8701=CARTESIAN_POINT ( 'NONE',  ( -41.00000000000000711, 53.00000000000000711, -38.50000000000000711 ) ) ;
#8704=DIRECTION ( 'NONE',  ( 0.000000000000000000, 0.000000000000000000, 1.000000000000000000 ) ) ;
#8717=ORIENTED_EDGE ( 'NONE', *, *, #2186, .F. ) ;
#8720=LINE ( 'NONE', #2944, #1603 ) ;
#8726=VECTOR ( 'NONE', #3195, 1000.000000000000000 ) ;
#8731=LINE ( 'NONE', #5904, #3652 ) ;
#8740=EDGE_CURVE ( 'NONE', #14902, #17473, #17461, .T. ) ;
#8741=EDGE_CURVE ( 'NONE', #13505, #6660, #9999, .T. ) ;
#8750=CARTESIAN_POINT ( 'NONE',  ( -24.00000000000000000, 110.0000000000000000, -5.999999999999998224 ) ) ;
#8759=LINE ( 'NONE', #16029, #4903 ) ;
#8760=AXIS2_PLACEMENT_3D ( 'NONE', #3342, #15682, #2252 ) ;
#8761=ORIENTED_EDGE ( 'NONE', *, *, #4338, .T. ) ;
#8762=EDGE_CURVE ( 'NONE', #17252, #9239, #15117, .T. ) ;
#8783=ORIENTED_EDGE ( 'NONE', *, *, #16958, .T. ) ;
#8784=VERTEX_POINT ( 'NONE', #9133 ) ;
#8785=EDGE_CURVE ( 'NONE', #2835, #2239, #1786, .T. ) ;
#8790=ORIENTED_EDGE ( 'NONE', *, *, #10869, .T. ) ;
#8794=EDGE_CURVE ( 'NONE', #16792, #3171, #6014, .T. ) ;
#8804=VERTEX_POINT ( 'NONE', #4833 ) ;
#8806=LINE ( 'NONE', #8701, #15632 ) ;
#8811=EDGE_CURVE ( 'NONE', #1380, #19125, #15016, .T. ) ;
#8812=FACE_OUTER_BOUND ( 'NONE', #3929, .T. ) ;
#8816=ORIENTED_EDGE ( 'NONE', *, *, #18058, .F. ) ;
#8827=ORIENTED_EDGE ( 'NONE', *, *, #3395, .T. ) ;
#8833=CARTESIAN_POINT ( 'NONE',  ( -24.00000000000000711, 53.00000000000000711, -25.50000000000000000 ) ) ;
#8835=PLANE ( 'NONE',  #18523 ) ;
#8846=CARTESIAN_POINT ( 'NONE',  ( -24.00000000000000000, 110.0000000000000000, -32.00000000000000000 ) ) ;
#8848=DIRECTION ( 'NONE',  ( 0.000000000000000000, 0.000000000000000000, 1.000000000000000000 ) ) ;
#8850=CARTESIAN_POINT ( 'NONE',  ( -24.00000000000000000, 110.0000000000000000, -12.49999999999999645 ) ) ;
#8855=DIRECTION ( 'NONE',  ( 1.000000000000000000, -0.000000000000000000, -0.000000000000000000 ) ) ;
#8856=DIRECTION ( 'NONE',  ( -1.000000000000000000, 0.000000000000000000, -0.000000000000000000 ) ) ;
#8861=DIRECTION ( 'NONE',  ( 0.000000000000000000, 0.000000000000000000, -1.000000000000000000 ) ) ;
#8879=EDGE_CURVE ( 'NONE', #13949, #3613, #9028, .T. ) ;
#8880=DIRECTION ( 'NONE',  ( 0.000000000000000000, 0.000000000000000000, -1.000000000000000000 ) ) ;
#8881=ORIENTED_EDGE ( 'NONE', *, *, #12064, .T. ) ;
#8885=DIRECTION ( 'NONE',  ( 0.000000000000000000, 0.000000000000000000, 1.000000000000000000 ) ) ;
#8898=EDGE_CURVE ( 'NONE', #18807, #14701, #15218, .T. ) ;
#8902=DIRECTION ( 'NONE',  ( 1.000000000000000000, -0.000000000000000000, -0.000000000000000000 ) ) ;
#8903=EDGE_CURVE ( 'NONE', #14415, #18998, #18264, .T. ) ;
#8906=CARTESIAN_POINT ( 'NONE',  ( -40.00000000000000711, 110.0000000000000000, -12.49999999999999645 ) ) ;
#8911=LINE ( 'NONE', #13314, #17747 ) ;
#8912=EDGE_LOOP ( 'NONE', ( #487, #13091, #17146, #707 ) ) ;
#8921=ORIENTED_EDGE ( 'NONE', *, *, #2452, .F. ) ;
#8928=CARTESIAN_POINT ( 'NONE',  ( -24.00000000000000000, 53.00000000000000711, 30.00000000000000000 ) ) ;
#8939=ADVANCED_FACE ( 'NONE', ( #8066 ), #15503, .F. ) ;
#8947=DIRECTION ( 'NONE',  ( 1.000000000000000000, -0.000000000000000000, -0.000000000000000000 ) ) ;
#8948=DIRECTION ( 'NONE',  ( 0.000000000000000000, 1.000000000000000000, 0.000000000000000000 ) ) ;
#8954=AXIS2_PLACEMENT_3D ( 'NONE', #6031, #16811, #13861 ) ;
#8966=VECTOR ( 'NONE', #16987, 1000.000000000000000 ) ;
#8971=CARTESIAN_POINT ( 'NONE',  ( -41.00000000000000711, 113.0000000000000000, 30.00000000000000000 ) ) ;
#8976=DIRECTION ( 'NONE',  ( -1.000000000000000000, 0.000000000000000000, 0.000000000000000000 ) ) ;
#8980=ORIENTED_EDGE ( 'NONE', *, *, #16453, .T. ) ;
#8984=DIRECTION ( 'NONE',  ( 1.000000000000000000, -0.000000000000000000, -0.000000000000000000 ) ) ;
#8993=ORIENTED_EDGE ( 'NONE', *, *, #13088, .F. ) ;
#8994=EDGE_CURVE ( 'NONE', #9118, #14005, #2166, .T. ) ;
#8995=EDGE_CURVE ( 'NONE', #8015, #16369, #14220, .T. ) ;
#9011=ORIENTED_EDGE ( 'NONE', *, *, #15306, .T. ) ;
#9020=ORIENTED_EDGE ( 'NONE', *, *, #13706, .T. ) ;
#9023=EDGE_CURVE ( 'NONE', #7944, #7050, #17168, .T. ) ;
#9026=DIRECTION ( 'NONE',  ( -1.000000000000000000, 0.000000000000000000, -0.000000000000000000 ) ) ;
#9028=LINE ( 'NONE', #13539, #16986 ) ;
#9044=CARTESIAN_POINT ( 'NONE',  ( -41.00000000000000711, 110.0000000000000000, 13.50000000000000000 ) ) ;
#9047=ORIENTED_EDGE ( 'NONE', *, *, #13917, .T. ) ;
#9053=EDGE_CURVE ( 'NONE', #9118, #7333, #13838, .T. ) ;
#9056=CARTESIAN_POINT ( 'NONE',  ( -24.00000000000000000, 113.0000000000000000, -50.00000000000000000 ) ) ;
#9057=VECTOR ( 'NONE', #9147, 1000.000000000000000 ) ;
#9059=ORIENTED_EDGE ( 'NONE', *, *, #2404, .F. ) ;
#9065=VECTOR ( 'NONE', #11900, 1000.000000000000000 ) ;
#9066=LINE ( 'NONE', #1631, #2266 ) ;
#9077=EDGE_CURVE ( 'NONE', #9, #16792, #12457, .T. ) ;
#9083=ORIENTED_EDGE ( 'NONE', *, *, #18834, .F. ) ;
#9084=ORIENTED_EDGE ( 'NONE', *, *, #16958, .F. ) ;
#9087=ORIENTED_EDGE ( 'NONE', *, *, #11983, .T. ) ;
#9090=DIRECTION ( 'NONE',  ( 0.000000000000000000, 0.000000000000000000, -1.000000000000000000 ) ) ;
#9106=VERTEX_POINT ( 'NONE', #5127 ) ;
#9113=ORIENTED_EDGE ( 'NONE', *, *, #18416, .F. ) ;
#9117=LINE ( 'NONE', #3139, #9383 ) ;
#9118=VERTEX_POINT ( 'NONE', #11080 ) ;
#9123=ORIENTED_EDGE ( 'NONE', *, *, #9299, .T. ) ;
#9129=LINE ( 'NONE', #8928, #9733 ) ;
#9133=CARTESIAN_POINT ( 'NONE',  ( -25.00000000000000711, 53.00000000000000711, -44.00000000000000000 ) ) ;
#9139=CARTESIAN_POINT ( 'NONE',  ( -40.00000000000000711, 110.0000000000000000, -37.50000000000000711 ) ) ;
#9146=ORIENTED_EDGE ( 'NONE', *, *, #7714, .F. ) ;
#9147=DIRECTION ( 'NONE',  ( 1.000000000000000000, -0.000000000000000000, -0.000000000000000000 ) ) ;
#9148=ORIENTED_EDGE ( 'NONE', *, *, #9455, .T. ) ;
#9156=DIRECTION ( 'NONE',  ( 0.000000000000000000, -1.000000000000000000, 0.000000000000000000 ) ) ;
#9176=CARTESIAN_POINT ( 'NONE',  ( -41.00000000000000711, 53.00000000000000711, 21.00000000000000000 ) ) ;
#9178=CARTESIAN_POINT ( 'NONE',  ( -41.00000000000000711, 53.00000000000000711, -6.000000000000001776 ) ) ;
#9180=ORIENTED_EDGE ( 'NONE', *, *, #17190, .F. ) ;
#9182=PRODUCT_DEFINITION ( 'UNKNOWN', '', #9237, #11576 ) ;
#9196=CARTESIAN_POINT ( 'NONE',  ( -32.50000000000000000, 52.00000000000000711, 12.34999999999999964 ) ) ;
#9197=EDGE_LOOP ( 'NONE', ( #10815, #2459, #368, #12906, #6077, #3107, #10572, #14233 ) ) ;
#9203=ORIENTED_EDGE ( 'NONE', *, *, #2246, .T. ) ;
#9216=CARTESIAN_POINT ( 'NONE',  ( -40.00000000000000711, 113.0000000000000000, 14.50000000000000000 ) ) ;
#9218=CARTESIAN_POINT ( 'NONE',  ( -24.00000000000000000, 53.00000000000000711, -25.49999999999999645 ) ) ;
#9223=CARTESIAN_POINT ( 'NONE',  ( -40.00000000000000711, 110.0000000000000000, -44.00000000000000000 ) ) ;
#9224=PLANE ( 'NONE',  #17417 ) ;
#9230=ORIENTED_EDGE ( 'NONE', *, *, #7832, .F. ) ;
#9232=CARTESIAN_POINT ( 'NONE',  ( -25.00000000000000000, 53.00000000000000711, 27.50000000000000000 ) ) ;
#9235=DIRECTION ( 'NONE',  ( -0.000000000000000000, -0.000000000000000000, -1.000000000000000000 ) ) ;
#9237=PRODUCT_DEFINITION_FORMATION_WITH_SPECIFIED_SOURCE ( 'ANY', '', #12997, .NOT_KNOWN. ) ;
#9238=PLANE ( 'NONE',  #342 ) ;
#9239=VERTEX_POINT ( 'NONE', #978 ) ;
#9241=FACE_OUTER_BOUND ( 'NONE', #49, .T. ) ;
#9244=EDGE_CURVE ( 'NONE', #9, #1049, #18185, .T. ) ;
#9247=LINE ( 'NONE', #1804, #4083 ) ;
#9249=DIRECTION ( 'NONE',  ( 0.000000000000000000, -1.000000000000000000, 0.000000000000000000 ) ) ;
#9250=CARTESIAN_POINT ( 'NONE',  ( -25.00000000000000000, 110.0000000000000000, 30.00000000000000000 ) ) ;
#9262=CARTESIAN_POINT ( 'NONE',  ( -41.00000000000000711, 53.00000000000000711, 6.999999999999999112 ) ) ;
#9267=VECTOR ( 'NONE', #11991, 1000.000000000000000 ) ;
#9269=CARTESIAN_POINT ( 'NONE',  ( -25.00000000000000000, 53.00000000000000711, 0.5000000000000004441 ) ) ;
#9274=VERTEX_POINT ( 'NONE', #17634 ) ;
#9283=LINE ( 'NONE', #14085, #802 ) ;
#9288=ORIENTED_EDGE ( 'NONE', *, *, #13331, .F. ) ;
#9290=LINE ( 'NONE', #379, #15038 ) ;
#9298=CARTESIAN_POINT ( 'NONE',  ( -41.00000000000000711, 53.00000000000000711, -18.00000000000000000 ) ) ;
#9299=EDGE_CURVE ( 'NONE', #5693, #12613, #2354, .T. ) ;
#9305=ORIENTED_EDGE ( 'NONE', *, *, #13803, .F. ) ;
#9339=CARTESIAN_POINT ( 'NONE',  ( -25.00000000000000000, 53.00000000000000711, 13.49999999999999822 ) ) ;
#9357=LINE ( 'NONE', #1926, #10059 ) ;
#9362=CARTESIAN_POINT ( 'NONE',  ( -25.00000000000000000, 53.00000000000000711, 30.00000000000000000 ) ) ;
#9364=CARTESIAN_POINT ( 'NONE',  ( -41.00000000000000711, 53.00000000000000711, 1.500000000000001332 ) ) ;
#9366=VERTEX_POINT ( 'NONE', #5976 ) ;
#9371=EDGE_LOOP ( 'NONE', ( #17436, #18243, #1312, #14897 ) ) ;
#9375=VECTOR ( 'NONE', #9438, 1000.000000000000000 ) ;
#9376=AXIS2_PLACEMENT_3D ( 'NONE', #2162, #11254, #13925 ) ;
#9383=VECTOR ( 'NONE', #7450, 1000.000000000000000 ) ;
#9392=VECTOR ( 'NONE', #778, 1000.000000000000000 ) ;
#9394=ORIENTED_EDGE ( 'NONE', *, *, #10257, .F. ) ;
#9395=ORIENTED_EDGE ( 'NONE', *, *, #15403, .T. ) ;
#9398=CIRCLE ( 'NONE', #12221, 2.649999999999985700 ) ;
#9399=ORIENTED_EDGE ( 'NONE', *, *, #5886, .F. ) ;
#9405=VERTEX_POINT ( 'NONE', #16460 ) ;
#9410=ORIENTED_EDGE ( 'NONE', *, *, #9457, .F. ) ;
#9412=EDGE_CURVE ( 'NONE', #4107, #12989, #18035, .T. ) ;
#9423=VECTOR ( 'NONE', #4532, 1000.000000000000000 ) ;
#9424=FACE_OUTER_BOUND ( 'NONE', #11838, .T. ) ;
#9436=VERTEX_POINT ( 'NONE', #16557 ) ;
#9438=DIRECTION ( 'NONE',  ( 0.000000000000000000, 0.000000000000000000, 1.000000000000000000 ) ) ;
#9439=VERTEX_POINT ( 'NONE', #7743 ) ;
#9442=PLANE ( 'NONE',  #790 ) ;
#9447=CARTESIAN_POINT ( 'NONE',  ( -41.00000000000000711, 110.0000000000000000, 1.500000000000001332 ) ) ;
#9448=CARTESIAN_POINT ( 'NONE',  ( -25.00000000000000711, 110.0000000000000000, -45.00000000000000000 ) ) ;
#9450=ORIENTED_EDGE ( 'NONE', *, *, #15414, .F. ) ;
#9455=EDGE_CURVE ( 'NONE', #14710, #17642, #15094, .T. ) ;
#9457=EDGE_CURVE ( 'NONE', #16369, #1200, #12137, .T. ) ;
#9466=CARTESIAN_POINT ( 'NONE',  ( -25.00000000000000000, 53.00000000000000711, 14.50000000000000000 ) ) ;
#9468=CARTESIAN_POINT ( 'NONE',  ( -25.00000000000000000, 110.0000000000000000, -24.49999999999999289 ) ) ;
#9476=EDGE_CURVE ( 'NONE', #14701, #185, #12237, .T. ) ;
#9481=ORIENTED_EDGE ( 'NONE', *, *, #5557, .F. ) ;
#9494=ORIENTED_EDGE ( 'NONE', *, *, #17300, .F. ) ;
#9501=FACE_OUTER_BOUND ( 'NONE', #16440, .T. ) ;
#9512=FACE_BOUND ( 'NONE', #6890, .T. ) ;
#9513=LINE ( 'NONE', #8153, #1608 ) ;
#9515=CARTESIAN_POINT ( 'NONE',  ( -25.00000000000000000, 53.00000000000000711, -19.00000000000000355 ) ) ;
#9516=DIRECTION ( 'NONE',  ( 1.000000000000000000, -0.000000000000000000, -0.000000000000000000 ) ) ;
#9518=FACE_OUTER_BOUND ( 'NONE', #16182, .T. ) ;
#9525=ADVANCED_FACE ( 'NONE', ( #8812 ), #14799, .T. ) ;
#9529=DIRECTION ( 'NONE',  ( -0.000000000000000000, -0.000000000000000000, -1.000000000000000000 ) ) ;
#9532=EDGE_CURVE ( 'NONE', #15030, #12335, #1468, .T. ) ;
#9534=CARTESIAN_POINT ( 'NONE',  ( -41.00000000000000711, 110.0000000000000000, 13.50000000000000000 ) ) ;
#9537=DIRECTION ( 'NONE',  ( 0.000000000000000000, 0.000000000000000000, -1.000000000000000000 ) ) ;
#9544=VECTOR ( 'NONE', #3562, 1000.000000000000000 ) ;
#9548=EDGE_CURVE ( 'NONE', #15895, #12743, #8227, .T. ) ;
#9567=VECTOR ( 'NONE', #8228, 1000.000000000000000 ) ;
#9570=CARTESIAN_POINT ( 'NONE',  ( -41.00000000000000711, 113.0000000000000000, 30.00000000000000000 ) ) ;
#9574=CARTESIAN_POINT ( 'NONE',  ( -24.00000000000000711, 110.0000000000000000, 1.500000000000001332 ) ) ;
#9576=CARTESIAN_POINT ( 'NONE',  ( -25.00000000000000711, 53.00000000000000711, 27.50000000000000000 ) ) ;
#9579=VECTOR ( 'NONE', #17766, 1000.000000000000000 ) ;
#9587=VERTEX_POINT ( 'NONE', #18617 ) ;
#9591=EDGE_CURVE ( 'NONE', #7475, #4404, #478, .T. ) ;
#9600=LINE ( 'NONE', #9216, #1911 ) ;
#9601=ORIENTED_EDGE ( 'NONE', *, *, #2055, .T. ) ;
#9602=AXIS2_PLACEMENT_3D ( 'NONE', #9176, #15161, #7711 ) ;
#9604=VERTEX_POINT ( 'NONE', #10758 ) ;
#9607=CARTESIAN_POINT ( 'NONE',  ( -40.00000000000000711, 53.00000000000000711, -30.99999999999999645 ) ) ;
#9608=EDGE_CURVE ( 'NONE', #4790, #19215, #12622, .T. ) ;
#9612=LINE ( 'NONE', #15598, #4610 ) ;
#9618=DIRECTION ( 'NONE',  ( 1.000000000000000000, -0.000000000000000000, -0.000000000000000000 ) ) ;
#9626=ORIENTED_EDGE ( 'NONE', *, *, #3470, .F. ) ;
#9635=DIRECTION ( 'NONE',  ( -0.000000000000000000, -0.000000000000000000, -1.000000000000000000 ) ) ;
#9647=LINE ( 'NONE', #10828, #1215 ) ;
#9649=EDGE_CURVE ( 'NONE', #12041, #1793, #5183, .T. ) ;
#9654=DIRECTION ( 'NONE',  ( 1.000000000000000000, -0.000000000000000000, -0.000000000000000000 ) ) ;
#9655=VECTOR ( 'NONE', #6145, 1000.000000000000000 ) ;
#9656=ORIENTED_EDGE ( 'NONE', *, *, #13067, .T. ) ;
#9661=FACE_OUTER_BOUND ( 'NONE', #14391, .T. ) ;
#9666=ORIENTED_EDGE ( 'NONE', *, *, #3097, .T. ) ;
#9670=EDGE_CURVE ( 'NONE', #76, #19248, #5097, .T. ) ;
#9695=LINE ( 'NONE', #14489, #7842 ) ;
#9703=CARTESIAN_POINT ( 'NONE',  ( -41.00000000000000711, 53.00000000000000711, 8.000000000000000000 ) ) ;
#9704=FACE_OUTER_BOUND ( 'NONE', #15359, .T. ) ;
#9710=LINE ( 'NONE', #8621, #17415 ) ;
#9716=DIRECTION ( 'NONE',  ( 1.000000000000000000, -0.000000000000000000, -0.000000000000000000 ) ) ;
#9720=CARTESIAN_POINT ( 'NONE',  ( -25.00000000000000000, 110.0000000000000000, 30.00000000000000000 ) ) ;
#9722=DIRECTION ( 'NONE',  ( 0.000000000000000000, 0.000000000000000000, -1.000000000000000000 ) ) ;
#9724=LINE ( 'NONE', #7891, #16319 ) ;
#9728=LINE ( 'NONE', #695, #18212 ) ;
#9732=EDGE_LOOP ( 'NONE', ( #6931, #4109, #4313, #7284 ) ) ;
#9733=VECTOR ( 'NONE', #12062, 1000.000000000000000 ) ;
#9738=EDGE_CURVE ( 'NONE', #2289, #9106, #11420, .T. ) ;
#9746=DIRECTION ( 'NONE',  ( 1.000000000000000000, -0.000000000000000000, -0.000000000000000000 ) ) ;
#9754=VECTOR ( 'NONE', #10158, 1000.000000000000000 ) ;
#9760=EDGE_CURVE ( 'NONE', #10640, #17050, #19082, .T. ) ;
#9762=ORIENTED_EDGE ( 'NONE', *, *, #14302, .T. ) ;
#9763=VECTOR ( 'NONE', #7904, 1000.000000000000000 ) ;
#9775=ORIENTED_EDGE ( 'NONE', *, *, #6928, .F. ) ;
#9787=DIRECTION ( 'NONE',  ( 0.000000000000000000, 0.000000000000000000, -1.000000000000000000 ) ) ;
#9788=ORIENTED_EDGE ( 'NONE', *, *, #2832, .F. ) ;
#9809=DIRECTION ( 'NONE',  ( 0.000000000000000000, 0.000000000000000000, -1.000000000000000000 ) ) ;
#9810=VERTEX_POINT ( 'NONE', #5653 ) ;
#9813=DIRECTION ( 'NONE',  ( 1.000000000000000000, -0.000000000000000000, -0.000000000000000000 ) ) ;
#9814=FACE_BOUND ( 'NONE', #14601, .T. ) ;
#9818=EDGE_LOOP ( 'NONE', ( #17445, #16273 ) ) ;
#9829=DIRECTION ( 'NONE',  ( -0.000000000000000000, -0.000000000000000000, -1.000000000000000000 ) ) ;
#9831=CARTESIAN_POINT ( 'NONE',  ( -41.00000000000000711, 110.0000000000000000, -37.50000000000000711 ) ) ;
#9834=LINE ( 'NONE', #17212, #17471 ) ;
#9835=CARTESIAN_POINT ( 'NONE',  ( -40.00000000000000711, 113.0000000000000000, -19.00000000000000355 ) ) ;
#9847=EDGE_CURVE ( 'NONE', #18913, #6733, #11617, .T. ) ;
#9877=ORIENTED_EDGE ( 'NONE', *, *, #5730, .T. ) ;
#9886=EDGE_CURVE ( 'NONE', #17827, #7050, #19182, .T. ) ;
#9891=EDGE_LOOP ( 'NONE', ( #18255, #16840, #10056, #6497 ) ) ;
#9907=VECTOR ( 'NONE', #1075, 1000.000000000000000 ) ;
#9913=ORIENTED_EDGE ( 'NONE', *, *, #760, .T. ) ;
#9917=LINE ( 'NONE', #11484, #14402 ) ;
#9929=CARTESIAN_POINT ( 'NONE',  ( -40.00000000000000711, 110.0000000000000000, 30.00000000000000000 ) ) ;
#9934=CARTESIAN_POINT ( 'NONE',  ( -41.00000000000000711, 53.00000000000000711, -11.50000000000000000 ) ) ;
#9948=ORIENTED_EDGE ( 'NONE', *, *, #13297, .T. ) ;
#9971=ADVANCED_FACE ( 'NONE', ( #4678 ), #7217, .T. ) ;
#9980=DIRECTION ( 'NONE',  ( 1.000000000000000000, 0.000000000000000000, 0.000000000000000000 ) ) ;
#9990=ORIENTED_EDGE ( 'NONE', *, *, #1295, .F. ) ;
#9992=DIRECTION ( 'NONE',  ( 0.000000000000000000, -1.000000000000000000, -0.000000000000000000 ) ) ;
#9994=DIRECTION ( 'NONE',  ( 0.000000000000000000, -1.000000000000000000, 0.000000000000000000 ) ) ;
#9999=LINE ( 'NONE', #3681, #16966 ) ;
#10006=ORIENTED_EDGE ( 'NONE', *, *, #11409, .F. ) ;
#10019=FACE_OUTER_BOUND ( 'NONE', #906, .T. ) ;
#10031=VECTOR ( 'NONE', #6223, 1000.000000000000000 ) ;
#10044=AXIS2_PLACEMENT_3D ( 'NONE', #14661, #17912, #1233 ) ;
#10048=DIRECTION ( 'NONE',  ( -1.156482317317871478E-16, 1.000000000000000000, 0.000000000000000000 ) ) ;
#10049=CARTESIAN_POINT ( 'NONE',  ( -40.00000000000000711, 110.0000000000000000, 30.00000000000000000 ) ) ;
#10051=VERTEX_POINT ( 'NONE', #437 ) ;
#10054=VERTEX_POINT ( 'NONE', #16905 ) ;
#10056=ORIENTED_EDGE ( 'NONE', *, *, #10236, .F. ) ;
#10059=VECTOR ( 'NONE', #5677, 1000.000000000000000 ) ;
#10066=ORIENTED_EDGE ( 'NONE', *, *, #1423, .F. ) ;
#10067=LINE ( 'NONE', #9262, #3589 ) ;
#10073=DIRECTION ( 'NONE',  ( -0.000000000000000000, 1.000000000000000000, -0.000000000000000000 ) ) ;
#10074=CARTESIAN_POINT ( 'NONE',  ( -41.00000000000000711, 110.0000000000000000, -18.00000000000000000 ) ) ;
#10077=ORIENTED_EDGE ( 'NONE', *, *, #10732, .T. ) ;
#10080=DIRECTION ( 'NONE',  ( 1.000000000000000000, -0.000000000000000000, -0.000000000000000000 ) ) ;
#10082=EDGE_CURVE ( 'NONE', #7137, #7631, #14050, .T. ) ;
#10084=EDGE_CURVE ( 'NONE', #16683, #9604, #15437, .T. ) ;
#10090=CARTESIAN_POINT ( 'NONE',  ( -40.00000000000000000, 53.00000000000000711, 30.00000000000000000 ) ) ;
#10091=VERTEX_POINT ( 'NONE', #13956 ) ;
#10094=CARTESIAN_POINT ( 'NONE',  ( -41.00000000000000711, 110.0000000000000000, 0.5000000000000004441 ) ) ;
#10098=FACE_BOUND ( 'NONE', #7345, .T. ) ;
#10102=EDGE_LOOP ( 'NONE', ( #8603, #17081, #9656, #7028 ) ) ;
#10109=ORIENTED_EDGE ( 'NONE', *, *, #4837, .F. ) ;
#10112=PLANE ( 'NONE',  #5471 ) ;
#10118=EDGE_CURVE ( 'NONE', #13021, #7331, #18288, .T. ) ;
#10121=DIRECTION ( 'NONE',  ( 0.000000000000000000, -1.000000000000000000, 0.000000000000000000 ) ) ;
#10122=ORIENTED_EDGE ( 'NONE', *, *, #5557, .T. ) ;
#10132=DIRECTION ( 'NONE',  ( 1.000000000000000000, -0.000000000000000000, -0.000000000000000000 ) ) ;
#10141=ORIENTED_EDGE ( 'NONE', *, *, #10118, .F. ) ;
#10145=ORIENTED_EDGE ( 'NONE', *, *, #8174, .T. ) ;
#10153=CARTESIAN_POINT ( 'NONE',  ( -41.00000000000000711, 110.0000000000000000, -37.50000000000000711 ) ) ;
#10158=DIRECTION ( 'NONE',  ( -0.000000000000000000, -0.000000000000000000, -1.000000000000000000 ) ) ;
#10162=CARTESIAN_POINT ( 'NONE',  ( -24.00000000000000000, 53.00000000000000711, -24.49999999999999289 ) ) ;
#10169=ORIENTED_EDGE ( 'NONE', *, *, #17800, .T. ) ;
#10174=ORIENTED_EDGE ( 'NONE', *, *, #6964, .T. ) ;
#10182=AXIS2_PLACEMENT_3D ( 'NONE', #19085, #8880, #10245 ) ;
#10183=LINE ( 'NONE', #19324, #8475 ) ;
#10194=ADVANCED_FACE ( 'NONE', ( #15724 ), #3852, .T. ) ;
#10196=FACE_OUTER_BOUND ( 'NONE', #19312, .T. ) ;
#10227=ORIENTED_EDGE ( 'NONE', *, *, #19263, .T. ) ;
#10236=EDGE_CURVE ( 'NONE', #2028, #8784, #722, .T. ) ;
#10245=DIRECTION ( 'NONE',  ( -1.000000000000000000, 0.000000000000000000, -0.000000000000000000 ) ) ;
#10251=VERTEX_POINT ( 'NONE', #18672 ) ;
#10257=EDGE_CURVE ( 'NONE', #15240, #17638, #9728, .T. ) ;
#10260=ORIENTED_EDGE ( 'NONE', *, *, #12811, .T. ) ;
#10264=DIRECTION ( 'NONE',  ( 0.000000000000000000, 0.000000000000000000, 1.000000000000000000 ) ) ;
#10274=ORIENTED_EDGE ( 'NONE', *, *, #2574, .F. ) ;
#10277=CARTESIAN_POINT ( 'NONE',  ( -41.00000000000000711, 53.00000000000000711, 14.50000000000000000 ) ) ;
#10279=EDGE_LOOP ( 'NONE', ( #7181, #3720, #12717, #4840 ) ) ;
#10283=ORIENTED_EDGE ( 'NONE', *, *, #2574, .T. ) ;
#10285=VERTEX_POINT ( 'NONE', #12551 ) ;
#10286=LINE ( 'NONE', #4432, #5353 ) ;
#10288=VECTOR ( 'NONE', #8855, 1000.000000000000000 ) ;
#10289=CARTESIAN_POINT ( 'NONE',  ( -24.00000000000000711, 53.00000000000000711, -6.000000000000001776 ) ) ;
#10291=CARTESIAN_POINT ( 'NONE',  ( -41.00000000000000711, 53.00000000000000711, -30.99999999999999645 ) ) ;
#10297=VERTEX_POINT ( 'NONE', #18258 ) ;
#10313=CARTESIAN_POINT ( 'NONE',  ( -41.00000000000000711, 53.00000000000000711, 0.5000000000000004441 ) ) ;
#10320=DIRECTION ( 'NONE',  ( 1.000000000000000000, -0.000000000000000000, -0.000000000000000000 ) ) ;
#10338=DIRECTION ( 'NONE',  ( 0.000000000000000000, 1.000000000000000000, 0.000000000000000000 ) ) ;
#10343=VECTOR ( 'NONE', #10048, 1000.000000000000000 ) ;
#10353=ORIENTED_EDGE ( 'NONE', *, *, #4744, .T. ) ;
#10361=ORIENTED_EDGE ( 'NONE', *, *, #7940, .T. ) ;
#10362=ORIENTED_EDGE ( 'NONE', *, *, #9670, .T. ) ;
#10368=FACE_OUTER_BOUND ( 'NONE', #981, .T. ) ;
#10372=DIRECTION ( 'NONE',  ( 0.000000000000000000, 1.000000000000000000, 0.000000000000000000 ) ) ;
#10376=ORIENTED_EDGE ( 'NONE', *, *, #4554, .F. ) ;
#10380=VERTEX_POINT ( 'NONE', #13922 ) ;
#10383=CARTESIAN_POINT ( 'NONE',  ( -40.00000000000000711, 110.0000000000000000, 1.500000000000001332 ) ) ;
#10393=VECTOR ( 'NONE', #150, 1000.000000000000000 ) ;
#10394=CARTESIAN_POINT ( 'NONE',  ( -25.00000000000000000, 113.0000000000000000, -50.00000000000000000 ) ) ;
#10396=CARTESIAN_POINT ( 'NONE',  ( -24.00000000000000000, 53.00000000000000711, 14.50000000000000000 ) ) ;
#10415=CARTESIAN_POINT ( 'NONE',  ( -24.00000000000000000, 110.0000000000000000, -45.00000000000000000 ) ) ;
#10423=DIRECTION ( 'NONE',  ( -1.000000000000000000, 0.000000000000000000, -0.000000000000000000 ) ) ;
#10432=CARTESIAN_POINT ( 'NONE',  ( -25.00000000000000000, 53.00000000000000711, -37.50000000000000711 ) ) ;
#10433=LINE ( 'NONE', #8971, #2782 ) ;
#10435=CARTESIAN_POINT ( 'NONE',  ( -41.00000000000000711, 110.0000000000000000, -37.50000000000000711 ) ) ;
#10441=ORIENTED_EDGE ( 'NONE', *, *, #7119, .F. ) ;
#10444=ORIENTED_EDGE ( 'NONE', *, *, #2698, .T. ) ;
#10456=ORIENTED_EDGE ( 'NONE', *, *, #810, .T. ) ;
#10459=CARTESIAN_POINT ( 'NONE',  ( -40.00000000000000711, 113.0000000000000000, -11.49999999999999645 ) ) ;
#10462=CARTESIAN_POINT ( 'NONE',  ( -41.00000000000000711, 110.0000000000000000, -24.49999999999999645 ) ) ;
#10466=CARTESIAN_POINT ( 'NONE',  ( -40.00000000000000711, 110.0000000000000000, 30.00000000000000000 ) ) ;
#10470=ORIENTED_EDGE ( 'NONE', *, *, #10575, .T. ) ;
#10475=EDGE_LOOP ( 'NONE', ( #6271, #15670, #5688, #19282 ) ) ;
#10481=VERTEX_POINT ( 'NONE', #17531 ) ;
#10484=ORIENTED_EDGE ( 'NONE', *, *, #9847, .F. ) ;
#10489=LINE ( 'NONE', #15114, #6439 ) ;
#10497=ORIENTED_EDGE ( 'NONE', *, *, #3921, .F. ) ;
#10500=VECTOR ( 'NONE', #5715, 1000.000000000000000 ) ;
#10505=EDGE_LOOP ( 'NONE', ( #2034, #11774, #681, #16665 ) ) ;
#10506=CARTESIAN_POINT ( 'NONE',  ( -24.00000000000000000, 53.00000000000000711, -31.00000000000000000 ) ) ;
#10524=FACE_OUTER_BOUND ( 'NONE', #9732, .T. ) ;
#10527=VECTOR ( 'NONE', #19334, 1000.000000000000000 ) ;
#10535=DIRECTION ( 'NONE',  ( -0.000000000000000000, -0.000000000000000000, -1.000000000000000000 ) ) ;
#10536=EDGE_CURVE ( 'NONE', #6823, #18134, #1161, .T. ) ;
#10540=LINE ( 'NONE', #9364, #18358 ) ;
#10550=EDGE_LOOP ( 'NONE', ( #11955, #12702, #14992, #5585 ) ) ;
#10566=CARTESIAN_POINT ( 'NONE',  ( -24.00000000000000711, 110.0000000000000000, 8.000000000000000000 ) ) ;
#10572=ORIENTED_EDGE ( 'NONE', *, *, #16555, .T. ) ;
#10575=EDGE_CURVE ( 'NONE', #5597, #12791, #14491, .T. ) ;
#10585=ORIENTED_EDGE ( 'NONE', *, *, #12173, .F. ) ;
#10597=EDGE_CURVE ( 'NONE', #9604, #7944, #3296, .T. ) ;
#10605=CARTESIAN_POINT ( 'NONE',  ( -41.00000000000000711, 53.00000000000000711, -18.00000000000000000 ) ) ;
#10609=DIRECTION ( 'NONE',  ( -1.000000000000000000, 0.000000000000000000, -0.000000000000000000 ) ) ;
#10613=DIRECTION ( 'NONE',  ( 0.000000000000000000, 0.000000000000000000, 1.000000000000000000 ) ) ;
#10617=EDGE_LOOP ( 'NONE', ( #4802, #16886, #10376, #8525, #8625, #11954, #6920, #16737 ) ) ;
#10625=CARTESIAN_POINT ( 'NONE',  ( -40.00000000000000711, 53.00000000000000711, -44.00000000000000000 ) ) ;
#10630=CARTESIAN_POINT ( 'NONE',  ( -25.00000000000000711, 53.00000000000000711, 21.00000000000000000 ) ) ;
#10632=LINE ( 'NONE', #16634, #1944 ) ;
#10636=FACE_OUTER_BOUND ( 'NONE', #13227, .T. ) ;
#10637=VECTOR ( 'NONE', #4478, 1000.000000000000000 ) ;
#10640=VERTEX_POINT ( 'NONE', #17727 ) ;
#10652=ORIENTED_EDGE ( 'NONE', *, *, #6126, .T. ) ;
#10653=ORIENTED_EDGE ( 'NONE', *, *, #11475, .F. ) ;
#10663=VECTOR ( 'NONE', #4726, 1000.000000000000000 ) ;
#10666=ORIENTED_EDGE ( 'NONE', *, *, #10236, .T. ) ;
#10670=VECTOR ( 'NONE', #4330, 1000.000000000000000 ) ;
#10672=ORIENTED_EDGE ( 'NONE', *, *, #8740, .T. ) ;
#10679=CYLINDRICAL_SURFACE ( 'NONE', #1253, 2.649999999999992806 ) ;
#10680=ORIENTED_EDGE ( 'NONE', *, *, #1634, .F. ) ;
#10688=FACE_BOUND ( 'NONE', #14726, .T. ) ;
#10732=EDGE_CURVE ( 'NONE', #6748, #18273, #9357, .T. ) ;
#10734=LINE ( 'NONE', #643, #4018 ) ;
#10735=DIRECTION ( 'NONE',  ( 1.000000000000000000, -0.000000000000000000, -0.000000000000000000 ) ) ;
#10740=ORIENTED_EDGE ( 'NONE', *, *, #7940, .F. ) ;
#10756=CARTESIAN_POINT ( 'NONE',  ( -41.00000000000000711, 53.00000000000000711, 27.50000000000000000 ) ) ;
#10758=CARTESIAN_POINT ( 'NONE',  ( -25.00000000000000711, 53.00000000000000711, 13.50000000000000000 ) ) ;
#10759=ORIENTED_EDGE ( 'NONE', *, *, #4171, .F. ) ;
#10773=ORIENTED_EDGE ( 'NONE', *, *, #13911, .F. ) ;
#10783=CARTESIAN_POINT ( 'NONE',  ( -41.00000000000000711, 53.00000000000000711, 8.000000000000000000 ) ) ;
#10784=ADVANCED_FACE ( 'NONE', ( #13070 ), #934, .T. ) ;
#10790=ORIENTED_EDGE ( 'NONE', *, *, #3458, .T. ) ;
#10793=CARTESIAN_POINT ( 'NONE',  ( -40.00000000000000000, 53.00000000000000711, 26.50000000000000000 ) ) ;
#10794=VERTEX_POINT ( 'NONE', #15751 ) ;
#10802=VECTOR ( 'NONE', #15524, 1000.000000000000000 ) ;
#10803=CARTESIAN_POINT ( 'NONE',  ( -24.00000000000000000, 110.0000000000000000, 26.50000000000000000 ) ) ;
#10813=VECTOR ( 'NONE', #14691, 1000.000000000000000 ) ;
#10815=ORIENTED_EDGE ( 'NONE', *, *, #12064, .F. ) ;
#10824=EDGE_CURVE ( 'NONE', #15240, #13814, #2497, .T. ) ;
#10826=VECTOR ( 'NONE', #15533, 1000.000000000000000 ) ;
#10828=CARTESIAN_POINT ( 'NONE',  ( -25.00000000000000000, 53.00000000000000711, -45.00000000000000000 ) ) ;
#10830=VECTOR ( 'NONE', #10121, 1000.000000000000000 ) ;
#10837=CARTESIAN_POINT ( 'NONE',  ( -25.00000000000000000, 110.0000000000000000, 30.00000000000000000 ) ) ;
#10839=ORIENTED_EDGE ( 'NONE', *, *, #5886, .T. ) ;
#10847=ADVANCED_FACE ( 'NONE', ( #6820 ), #1034, .T. ) ;
#10848=DIRECTION ( 'NONE',  ( 0.000000000000000000, 1.000000000000000000, 0.000000000000000000 ) ) ;
#10854=LINE ( 'NONE', #16849, #15621 ) ;
#10855=CARTESIAN_POINT ( 'NONE',  ( -40.00000000000000711, 113.0000000000000000, 20.00000000000000000 ) ) ;
#10869=EDGE_CURVE ( 'NONE', #3171, #16792, #12883, .T. ) ;
#10877=ORIENTED_EDGE ( 'NONE', *, *, #19064, .F. ) ;
#10890=DIRECTION ( 'NONE',  ( 0.000000000000000000, 0.000000000000000000, -1.000000000000000000 ) ) ;
#10896=ADVANCED_FACE ( 'NONE', ( #10524 ), #4664, .F. ) ;
#10908=DIRECTION ( 'NONE',  ( -0.000000000000000000, 1.000000000000000000, -0.000000000000000000 ) ) ;
#10912=ORIENTED_EDGE ( 'NONE', *, *, #8994, .F. ) ;
#10921=VECTOR ( 'NONE', #11535, 1000.000000000000000 ) ;
#10928=CARTESIAN_POINT ( 'NONE',  ( -25.00000000000000000, 53.00000000000000711, -50.00000000000000000 ) ) ;
#10932=ORIENTED_EDGE ( 'NONE', *, *, #19039, .T. ) ;
#10940=DIRECTION ( 'NONE',  ( 0.000000000000000000, 0.000000000000000000, -1.000000000000000000 ) ) ;
#10943=VECTOR ( 'NONE', #18732, 1000.000000000000000 ) ;
#10947=VERTEX_POINT ( 'NONE', #8846 ) ;
#10968=PLANE ( 'NONE',  #630 ) ;
#10974=DIRECTION ( 'NONE',  ( 0.000000000000000000, -1.000000000000000000, 0.000000000000000000 ) ) ;
#10976=DIRECTION ( 'NONE',  ( 1.000000000000000000, -0.000000000000000000, -0.000000000000000000 ) ) ;
#10978=CARTESIAN_POINT ( 'NONE',  ( -24.00000000000000711, 110.0000000000000000, 21.00000000000000000 ) ) ;
#10988=ORIENTED_EDGE ( 'NONE', *, *, #15306, .F. ) ;
#10991=VECTOR ( 'NONE', #16138, 1000.000000000000000 ) ;
#10992=DIRECTION ( 'NONE',  ( 0.000000000000000000, 0.000000000000000000, 1.000000000000000000 ) ) ;
#10993=ORIENTED_EDGE ( 'NONE', *, *, #14966, .T. ) ;
#11001=ORIENTED_EDGE ( 'NONE', *, *, #2569, .T. ) ;
#11004=VECTOR ( 'NONE', #1725, 1000.000000000000000 ) ;
#11005=CARTESIAN_POINT ( 'NONE',  ( -41.00000000000000711, 110.0000000000000000, -45.00000000000000000 ) ) ;
#11007=LINE ( 'NONE', #17008, #1705 ) ;
#11009=CARTESIAN_POINT ( 'NONE',  ( 0.000000000000000000, 0.000000000000000000, -50.00000000000000000 ) ) ;
#11010=CARTESIAN_POINT ( 'NONE',  ( -41.00000000000000711, 110.0000000000000000, -32.00000000000000000 ) ) ;
#11011=VECTOR ( 'NONE', #3152, 1000.000000000000000 ) ;
#11017=FACE_OUTER_BOUND ( 'NONE', #17552, .T. ) ;
#11019=CARTESIAN_POINT ( 'NONE',  ( -40.00000000000000711, 113.0000000000000000, -5.000000000000004441 ) ) ;
#11024=CARTESIAN_POINT ( 'NONE',  ( -41.00000000000000711, 53.00000000000000711, -5.000000000000000888 ) ) ;
#11026=CARTESIAN_POINT ( 'NONE',  ( -41.00000000000000711, 53.00000000000000711, -37.50000000000000711 ) ) ;
#11030=DIRECTION ( 'NONE',  ( 0.000000000000000000, 1.000000000000000000, 0.000000000000000000 ) ) ;
#11034=EDGE_CURVE ( 'NONE', #10794, #11529, #11242, .T. ) ;
#11038=CARTESIAN_POINT ( 'NONE',  ( -41.00000000000000711, 53.00000000000000711, 0.5000000000000004441 ) ) ;
#11064=PLANE ( 'NONE',  #8760 ) ;
#11069=EDGE_CURVE ( 'NONE', #10640, #2931, #15128, .T. ) ;
#11071=CARTESIAN_POINT ( 'NONE',  ( -24.00000000000000711, 53.00000000000000711, -24.49999999999999645 ) ) ;
#11076=FACE_BOUND ( 'NONE', #12314, .T. ) ;
#11080=CARTESIAN_POINT ( 'NONE',  ( -41.00000000000000711, 53.00000000000000711, -45.00000000000000000 ) ) ;
#11089=ADVANCED_BREP_SHAPE_REPRESENTATION ( '', ( #17097, #1791 ), #2707 ) ;
#11092=DIRECTION ( 'NONE',  ( 0.000000000000000000, 0.000000000000000000, 1.000000000000000000 ) ) ;
#11093=ORIENTED_EDGE ( 'NONE', *, *, #18361, .F. ) ;
#11095=ORIENTED_EDGE ( 'NONE', *, *, #5730, .F. ) ;
#11097=CARTESIAN_POINT ( 'NONE',  ( -25.00000000000000711, 53.00000000000000711, -5.000000000000000888 ) ) ;
#11099=LINE ( 'NONE', #9534, #668 ) ;
#11108=VECTOR ( 'NONE', #998, 1000.000000000000000 ) ;
#11112=DIRECTION ( 'NONE',  ( 0.000000000000000000, 1.000000000000000000, 0.000000000000000000 ) ) ;
#11123=LINE ( 'NONE', #17028, #7723 ) ;
#11130=PLANE ( 'NONE',  #12390 ) ;
#11133=VECTOR ( 'NONE', #10613, 1000.000000000000000 ) ;
#11151=ORIENTED_EDGE ( 'NONE', *, *, #6639, .F. ) ;
#11164=ORIENTED_EDGE ( 'NONE', *, *, #3136, .F. ) ;
#11175=CARTESIAN_POINT ( 'NONE',  ( -40.00000000000000000, 52.00000000000000711, -50.00000000000000000 ) ) ;
#11177=ORIENTED_EDGE ( 'NONE', *, *, #1250, .T. ) ;
#11183=LINE ( 'NONE', #18931, #13779 ) ;
#11185=LINE ( 'NONE', #8445, #16583 ) ;
#11187=FACE_OUTER_BOUND ( 'NONE', #6351, .T. ) ;
#11191=DIRECTION ( 'NONE',  ( 0.000000000000000000, 1.000000000000000000, 0.000000000000000000 ) ) ;
#11196=ORIENTED_EDGE ( 'NONE', *, *, #19178, .F. ) ;
#11202=FACE_OUTER_BOUND ( 'NONE', #1936, .T. ) ;
#11204=DIRECTION ( 'NONE',  ( 0.000000000000000000, -1.000000000000000000, -0.000000000000000000 ) ) ;
#11235=ORIENTED_EDGE ( 'NONE', *, *, #15123, .T. ) ;
#11237=ORIENTED_EDGE ( 'NONE', *, *, #9476, .F. ) ;
#11238=ORIENTED_EDGE ( 'NONE', *, *, #14652, .T. ) ;
#11241=AXIS2_PLACEMENT_3D ( 'NONE', #10153, #8602, #5570 ) ;
#11242=LINE ( 'NONE', #18542, #3201 ) ;
#11247=AXIS2_PLACEMENT_3D ( 'NONE', #17185, #9722, #14328 ) ;
#11249=VERTEX_POINT ( 'NONE', #12910 ) ;
#11251=ORIENTED_EDGE ( 'NONE', *, *, #17189, .F. ) ;
#11254=DIRECTION ( 'NONE',  ( 0.000000000000000000, 1.000000000000000000, 0.000000000000000000 ) ) ;
#11255=VECTOR ( 'NONE', #4429, 1000.000000000000000 ) ;
#11258=CARTESIAN_POINT ( 'NONE',  ( -41.00000000000000711, 53.00000000000000711, -45.00000000000000000 ) ) ;
#11260=DIRECTION ( 'NONE',  ( -0.000000000000000000, 1.000000000000000000, -0.000000000000000000 ) ) ;
#11280=CARTESIAN_POINT ( 'NONE',  ( -24.00000000000000000, 110.0000000000000000, -19.00000000000000355 ) ) ;
#11282=CARTESIAN_POINT ( 'NONE',  ( -41.00000000000000711, 53.00000000000000711, 20.00000000000000000 ) ) ;
#11286=ADVANCED_FACE ( 'NONE', ( #2524 ), #17620, .T. ) ;
#11293=VECTOR ( 'NONE', #18150, 1000.000000000000000 ) ;
#11294=ORIENTED_EDGE ( 'NONE', *, *, #1384, .F. ) ;
#11308=EDGE_CURVE ( 'NONE', #12927, #17827, #14483, .T. ) ;
#11320=DIRECTION ( 'NONE',  ( 0.000000000000000000, 0.000000000000000000, -1.000000000000000000 ) ) ;
#11327=PLANE ( 'NONE',  #1620 ) ;
#11330=DIRECTION ( 'NONE',  ( 0.000000000000000000, 0.000000000000000000, -1.000000000000000000 ) ) ;
#11337=SURFACE_STYLE_FILL_AREA ( #18996 ) ;
#11338=VERTEX_POINT ( 'NONE', #11934 ) ;
#11353=CARTESIAN_POINT ( 'NONE',  ( -25.00000000000000000, 110.0000000000000000, 30.00000000000000000 ) ) ;
#11367=FACE_OUTER_BOUND ( 'NONE', #6372, .T. ) ;
#11369=DIRECTION ( 'NONE',  ( 0.000000000000000000, 0.000000000000000000, 1.000000000000000000 ) ) ;
#11370=ORIENTED_EDGE ( 'NONE', *, *, #18991, .F. ) ;
#11398=DIRECTION ( 'NONE',  ( -0.000000000000000000, 1.000000000000000000, -0.000000000000000000 ) ) ;
#11402=ORIENTED_EDGE ( 'NONE', *, *, #4485, .F. ) ;
#11409=EDGE_CURVE ( 'NONE', #1646, #11598, #9066, .T. ) ;
#11412=ORIENTED_EDGE ( 'NONE', *, *, #16721, .F. ) ;
#11420=LINE ( 'NONE', #15944, #10991 ) ;
#11424=ORIENTED_EDGE ( 'NONE', *, *, #11976, .F. ) ;
#11425=EDGE_CURVE ( 'NONE', #18025, #185, #18198, .T. ) ;
#11438=ORIENTED_EDGE ( 'NONE', *, *, #6601, .T. ) ;
#11448=VECTOR ( 'NONE', #18597, 1000.000000000000000 ) ;
#11465=CARTESIAN_POINT ( 'NONE',  ( -41.00000000000000711, 110.0000000000000000, -37.50000000000000711 ) ) ;
#11469=DIRECTION ( 'NONE',  ( 0.000000000000000000, 1.000000000000000000, 0.000000000000000000 ) ) ;
#11474=FILL_AREA_STYLE_COLOUR ( '', #3574 ) ;
#11475=EDGE_CURVE ( 'NONE', #13021, #18278, #11907, .T. ) ;
#11484=CARTESIAN_POINT ( 'NONE',  ( -25.00000000000000000, 53.00000000000000711, 8.000000000000000000 ) ) ;
#11488=DIRECTION ( 'NONE',  ( -0.000000000000000000, 1.000000000000000000, 0.000000000000000000 ) ) ;
#11497=LINE ( 'NONE', #17893, #1759 ) ;
#11502=DIRECTION ( 'NONE',  ( 0.000000000000000000, 0.000000000000000000, -1.000000000000000000 ) ) ;
#11505=CARTESIAN_POINT ( 'NONE',  ( -40.00000000000000711, 113.0000000000000000, -44.00000000000000000 ) ) ;
#11508=DIRECTION ( 'NONE',  ( 0.000000000000000000, 0.000000000000000000, -1.000000000000000000 ) ) ;
#11509=VECTOR ( 'NONE', #6717, 1000.000000000000000 ) ;
#11513=EDGE_CURVE ( 'NONE', #7340, #12537, #1920, .T. ) ;
#11520=ORIENTED_EDGE ( 'NONE', *, *, #15511, .T. ) ;
#11526=DIRECTION ( 'NONE',  ( 0.000000000000000000, 1.000000000000000000, 0.000000000000000000 ) ) ;
#11529=VERTEX_POINT ( 'NONE', #15443 ) ;
#11532=FACE_OUTER_BOUND ( 'NONE', #17132, .T. ) ;
#11533=VERTEX_POINT ( 'NONE', #2009 ) ;
#11535=DIRECTION ( 'NONE',  ( 0.000000000000000000, 0.000000000000000000, -1.000000000000000000 ) ) ;
#11541=VECTOR ( 'NONE', #12845, 1000.000000000000000 ) ;
#11542=LINE ( 'NONE', #10074, #2991 ) ;
#11545=ORIENTED_EDGE ( 'NONE', *, *, #14988, .F. ) ;
#11548=EDGE_CURVE ( 'NONE', #993, #11714, #7999, .T. ) ;
#11551=ORIENTED_EDGE ( 'NONE', *, *, #9760, .T. ) ;
#11558=CARTESIAN_POINT ( 'NONE',  ( -32.50000000000000000, 52.00000000000000711, -32.35000000000000142 ) ) ;
#11560=CARTESIAN_POINT ( 'NONE',  ( -25.00000000000000711, 53.00000000000000711, -24.49999999999999645 ) ) ;
#11565=CARTESIAN_POINT ( 'NONE',  ( -41.00000000000000711, 110.0000000000000000, -30.99999999999999645 ) ) ;
#11566=VECTOR ( 'NONE', #6943, 1000.000000000000000 ) ;
#11570=FACE_BOUND ( 'NONE', #19131, .T. ) ;
#11573=VECTOR ( 'NONE', #18130, 1000.000000000000000 ) ;
#11576=PRODUCT_DEFINITION_CONTEXT ( 'detailed design', #6073, 'design' ) ;
#11593=VECTOR ( 'NONE', #3908, 1000.000000000000000 ) ;
#11597=VECTOR ( 'NONE', #14330, 1000.000000000000000 ) ;
#11598=VERTEX_POINT ( 'NONE', #17018 ) ;
#11611=DIRECTION ( 'NONE',  ( -1.000000000000000000, 0.000000000000000000, -0.000000000000000000 ) ) ;
#11612=ADVANCED_FACE ( 'NONE', ( #11017 ), #13769, .T. ) ;
#11617=LINE ( 'NONE', #4084, #10343 ) ;
#11620=ORIENTED_EDGE ( 'NONE', *, *, #13067, .F. ) ;
#11623=EDGE_CURVE ( 'NONE', #2609, #10285, #635, .T. ) ;
#11627=ORIENTED_EDGE ( 'NONE', *, *, #5467, .T. ) ;
#11633=DIRECTION ( 'NONE',  ( 0.000000000000000000, -1.000000000000000000, 0.000000000000000000 ) ) ;
#11637=EDGE_LOOP ( 'NONE', ( #5133, #16812, #10141, #1386 ) ) ;
#11638=ORIENTED_EDGE ( 'NONE', *, *, #2398, .T. ) ;
#11643=ADVANCED_FACE ( 'NONE', ( #349 ), #12680, .T. ) ;
#11645=DIRECTION ( 'NONE',  ( 0.000000000000000000, 0.000000000000000000, -1.000000000000000000 ) ) ;
#11649=EDGE_LOOP ( 'NONE', ( #18533, #14102, #15262, #1173 ) ) ;
#11652=VERTEX_POINT ( 'NONE', #17583 ) ;
#11673=CARTESIAN_POINT ( 'NONE',  ( -25.00000000000000000, 53.00000000000000711, -32.00000000000000000 ) ) ;
#11675=EDGE_CURVE ( 'NONE', #2269, #9366, #14442, .T. ) ;
#11682=LINE ( 'NONE', #7087, #17213 ) ;
#11684=LINE ( 'NONE', #5528, #15488 ) ;
#11692=FACE_BOUND ( 'NONE', #18653, .T. ) ;
#11694=LINE ( 'NONE', #17686, #5213 ) ;
#11695=EDGE_CURVE ( 'NONE', #3613, #5230, #11682, .T. ) ;
#11697=LINE ( 'NONE', #17990, #9065 ) ;
#11698=VECTOR ( 'NONE', #12670, 1000.000000000000000 ) ;
#11714=VERTEX_POINT ( 'NONE', #17298 ) ;
#11715=ORIENTED_EDGE ( 'NONE', *, *, #14861, .T. ) ;
#11719=ORIENTED_EDGE ( 'NONE', *, *, #11793, .F. ) ;
#11726=EDGE_LOOP ( 'NONE', ( #10109, #8666, #14666, #5870 ) ) ;
#11733=CARTESIAN_POINT ( 'NONE',  ( -40.00000000000000711, 113.0000000000000000, 27.50000000000000000 ) ) ;
#11738=VECTOR ( 'NONE', #6060, 1000.000000000000000 ) ;
#11757=LINE ( 'NONE', #17955, #4709 ) ;
#11760=PLANE ( 'NONE',  #19 ) ;
#11764=CARTESIAN_POINT ( 'NONE',  ( -41.00000000000000711, 53.00000000000000711, 1.500000000000001332 ) ) ;
#11768=CARTESIAN_POINT ( 'NONE',  ( -24.00000000000000711, 110.0000000000000000, 14.50000000000000000 ) ) ;
#11774=ORIENTED_EDGE ( 'NONE', *, *, #2404, .T. ) ;
#11785=CARTESIAN_POINT ( 'NONE',  ( -41.00000000000000711, 53.00000000000000711, 21.00000000000000000 ) ) ;
#11787=DIRECTION ( 'NONE',  ( 1.000000000000000000, -0.000000000000000000, -0.000000000000000000 ) ) ;
#11790=VECTOR ( 'NONE', #17307, 1000.000000000000000 ) ;
#11793=EDGE_CURVE ( 'NONE', #14672, #18913, #14342, .T. ) ;
#11806=DIRECTION ( 'NONE',  ( 0.000000000000000000, -1.000000000000000000, -0.000000000000000000 ) ) ;
#11808=DIRECTION ( 'NONE',  ( 1.000000000000000000, -0.000000000000000000, -0.000000000000000000 ) ) ;
#11811=CARTESIAN_POINT ( 'NONE',  ( -40.00000000000000711, 110.0000000000000000, 30.00000000000000000 ) ) ;
#11813=LINE ( 'NONE', #13280, #5512 ) ;
#11826=VERTEX_POINT ( 'NONE', #8850 ) ;
#11829=CARTESIAN_POINT ( 'NONE',  ( -41.00000000000000711, 53.00000000000000711, -37.50000000000000711 ) ) ;
#11838=EDGE_LOOP ( 'NONE', ( #7451, #1574, #3657, #4303 ) ) ;
#11839=VERTEX_POINT ( 'NONE', #17879 ) ;
#11842=AXIS2_PLACEMENT_3D ( 'NONE', #10313, #11888, #14740 ) ;
#11849=ORIENTED_EDGE ( 'NONE', *, *, #9023, .F. ) ;
#11852=DIRECTION ( 'NONE',  ( 0.000000000000000000, 0.000000000000000000, 1.000000000000000000 ) ) ;
#11859=DIRECTION ( 'NONE',  ( 0.000000000000000000, 0.000000000000000000, -1.000000000000000000 ) ) ;
#11862=DIRECTION ( 'NONE',  ( 1.000000000000000000, -0.000000000000000000, -0.000000000000000000 ) ) ;
#11866=PLANE ( 'NONE',  #6452 ) ;
#11878=CARTESIAN_POINT ( 'NONE',  ( -32.50000000000000000, 53.00000000000000711, -35.00000000000000000 ) ) ;
#11881=VECTOR ( 'NONE', #4821, 1000.000000000000000 ) ;
#11888=DIRECTION ( 'NONE',  ( 0.000000000000000000, 0.000000000000000000, -1.000000000000000000 ) ) ;
#11890=VECTOR ( 'NONE', #7933, 1000.000000000000000 ) ;
#11894=EDGE_CURVE ( 'NONE', #11839, #12989, #16202, .T. ) ;
#11900=DIRECTION ( 'NONE',  ( 0.000000000000000000, -1.000000000000000000, 0.000000000000000000 ) ) ;
#11902=CARTESIAN_POINT ( 'NONE',  ( -41.00000000000000711, 53.00000000000000711, -25.50000000000000000 ) ) ;
#11906=EDGE_CURVE ( 'NONE', #7234, #17473, #4549, .T. ) ;
#11907=LINE ( 'NONE', #5248, #15729 ) ;
#11914=CARTESIAN_POINT ( 'NONE',  ( -24.00000000000000711, 110.0000000000000000, -24.49999999999999645 ) ) ;
#11916=PLANE ( 'NONE',  #10044 ) ;
#11917=VECTOR ( 'NONE', #19035, 1000.000000000000000 ) ;
#11926=EDGE_LOOP ( 'NONE', ( #1314, #4340, #11959, #12531 ) ) ;
#11929=EDGE_CURVE ( 'NONE', #12743, #5230, #18077, .T. ) ;
#11934=CARTESIAN_POINT ( 'NONE',  ( -25.00000000000000000, 53.00000000000000711, 30.00000000000000000 ) ) ;
#11941=ORIENTED_EDGE ( 'NONE', *, *, #7715, .T. ) ;
#11947=CARTESIAN_POINT ( 'NONE',  ( -41.00000000000000711, 53.00000000000000711, -19.00000000000000000 ) ) ;
#11948=ORIENTED_EDGE ( 'NONE', *, *, #14966, .F. ) ;
#11954=ORIENTED_EDGE ( 'NONE', *, *, #3264, .F. ) ;
#11955=ORIENTED_EDGE ( 'NONE', *, *, #8652, .F. ) ;
#11959=ORIENTED_EDGE ( 'NONE', *, *, #12811, .F. ) ;
#11961=ORIENTED_EDGE ( 'NONE', *, *, #5180, .T. ) ;
#11963=EDGE_LOOP ( 'NONE', ( #7533, #4501, #5736, #15766 ) ) ;
#11967=DIRECTION ( 'NONE',  ( 0.000000000000000000, 0.000000000000000000, 1.000000000000000000 ) ) ;
#11976=EDGE_CURVE ( 'NONE', #12423, #1050, #18377, .T. ) ;
#11979=ORIENTED_EDGE ( 'NONE', *, *, #19083, .T. ) ;
#11983=EDGE_CURVE ( 'NONE', #8044, #7340, #14041, .T. ) ;
#11989=PLANE ( 'NONE',  #15165 ) ;
#11991=DIRECTION ( 'NONE',  ( 0.000000000000000000, -1.000000000000000000, 0.000000000000000000 ) ) ;
#12000=CARTESIAN_POINT ( 'NONE',  ( -40.00000000000000711, 110.0000000000000000, -45.00000000000000000 ) ) ;
#12004=LINE ( 'NONE', #7709, #4660 ) ;
#12009=EDGE_CURVE ( 'NONE', #1553, #6936, #4944, .T. ) ;
#12010=EDGE_CURVE ( 'NONE', #76, #3347, #3464, .T. ) ;
#12033=ORIENTED_EDGE ( 'NONE', *, *, #3458, .F. ) ;
#12041=VERTEX_POINT ( 'NONE', #2181 ) ;
#12042=ORIENTED_EDGE ( 'NONE', *, *, #10732, .F. ) ;
#12059=LINE ( 'NONE', #7660, #16619 ) ;
#12061=AXIS2_PLACEMENT_3D ( 'NONE', #16991, #601, #15220 ) ;
#12062=DIRECTION ( 'NONE',  ( 0.000000000000000000, 0.000000000000000000, -1.000000000000000000 ) ) ;
#12064=EDGE_CURVE ( 'NONE', #1874, #15591, #8171, .T. ) ;
#12066=CARTESIAN_POINT ( 'NONE',  ( -41.00000000000000711, 113.0000000000000000, -50.00000000000000000 ) ) ;
#12070=ORIENTED_EDGE ( 'NONE', *, *, #15140, .T. ) ;
#12114=VERTEX_POINT ( 'NONE', #17000 ) ;
#12132=ORIENTED_EDGE ( 'NONE', *, *, #11034, .F. ) ;
#12137=LINE ( 'NONE', #3027, #5644 ) ;
#12138=LINE ( 'NONE', #9298, #6139 ) ;
#12140=VERTEX_POINT ( 'NONE', #10803 ) ;
#12144=VERTEX_POINT ( 'NONE', #16799 ) ;
#12148=LINE ( 'NONE', #19321, #5946 ) ;
#12153=ADVANCED_FACE ( 'NONE', ( #9241 ), #15231, .F. ) ;
#12165=PLANE ( 'NONE',  #12061 ) ;
#12173=EDGE_CURVE ( 'NONE', #10794, #3796, #11185, .T. ) ;
#12178=ORIENTED_EDGE ( 'NONE', *, *, #1634, .T. ) ;
#12199=DIRECTION ( 'NONE',  ( 1.000000000000000000, -0.000000000000000000, -0.000000000000000000 ) ) ;
#12205=CARTESIAN_POINT ( 'NONE',  ( -41.00000000000000711, 53.00000000000000711, 0.5000000000000004441 ) ) ;
#12215=AXIS2_PLACEMENT_3D ( 'NONE', #412, #5300, #8251 ) ;
#12221=AXIS2_PLACEMENT_3D ( 'NONE', #11878, #17876, #8848 ) ;
#12224=ORIENTED_EDGE ( 'NONE', *, *, #10536, .T. ) ;
#12226=EDGE_CURVE ( 'NONE', #19128, #1572, #17183, .T. ) ;
#12233=CARTESIAN_POINT ( 'NONE',  ( -24.00000000000000711, 53.00000000000000711, -12.50000000000000000 ) ) ;
#12234=EDGE_CURVE ( 'NONE', #209, #9274, #7065, .T. ) ;
#12235=VECTOR ( 'NONE', #3328, 1000.000000000000000 ) ;
#12237=LINE ( 'NONE', #13606, #11573 ) ;
#12242=ORIENTED_EDGE ( 'NONE', *, *, #5806, .T. ) ;
#12249=EDGE_CURVE ( 'NONE', #2289, #18664, #6875, .T. ) ;
#12252=VECTOR ( 'NONE', #12671, 1000.000000000000000 ) ;
#12254=FACE_OUTER_BOUND ( 'NONE', #9371, .T. ) ;
#12255=ORIENTED_EDGE ( 'NONE', *, *, #8994, .T. ) ;
#12258=CARTESIAN_POINT ( 'NONE',  ( -24.00000000000000000, 110.0000000000000000, 30.00000000000000000 ) ) ;
#12259=ORIENTED_EDGE ( 'NONE', *, *, #17800, .F. ) ;
#12265=FACE_BOUND ( 'NONE', #230, .T. ) ;
#12268=CARTESIAN_POINT ( 'NONE',  ( -41.00000000000000711, 110.0000000000000000, -18.00000000000000000 ) ) ;
#12269=DIRECTION ( 'NONE',  ( 0.000000000000000000, 0.000000000000000000, 1.000000000000000000 ) ) ;
#12270=AXIS2_PLACEMENT_3D ( 'NONE', #12787, #5360, #11320 ) ;
#12272=DIRECTION ( 'NONE',  ( 0.000000000000000000, -1.000000000000000000, -0.000000000000000000 ) ) ;
#12273=ORIENTED_EDGE ( 'NONE', *, *, #10082, .F. ) ;
#12275=DIRECTION ( 'NONE',  ( 0.000000000000000000, 0.000000000000000000, 1.000000000000000000 ) ) ;
#12276=ADVANCED_FACE ( 'NONE', ( #19031 ), #15803, .T. ) ;
#12277=ORIENTED_EDGE ( 'NONE', *, *, #15152, .F. ) ;
#12283=AXIS2_PLACEMENT_3D ( 'NONE', #6335, #3575, #16820 ) ;
#12285=ORIENTED_EDGE ( 'NONE', *, *, #7715, .F. ) ;
#12286=ORIENTED_EDGE ( 'NONE', *, *, #2222, .T. ) ;
#12288=DIRECTION ( 'NONE',  ( 0.000000000000000000, 1.000000000000000000, 0.000000000000000000 ) ) ;
#12291=EDGE_CURVE ( 'NONE', #11714, #8784, #2458, .T. ) ;
#12293=EDGE_CURVE ( 'NONE', #9118, #4107, #1180, .T. ) ;
#12301=CARTESIAN_POINT ( 'NONE',  ( -41.00000000000000711, 53.00000000000000711, -18.00000000000000000 ) ) ;
#12314=EDGE_LOOP ( 'NONE', ( #7159, #6166, #15980, #4682 ) ) ;
#12325=ORIENTED_EDGE ( 'NONE', *, *, #3972, .T. ) ;
#12335=VERTEX_POINT ( 'NONE', #11560 ) ;
#12337=VERTEX_POINT ( 'NONE', #18666 ) ;
#12339=( LENGTH_UNIT ( ) NAMED_UNIT ( * ) SI_UNIT ( .MILLI., .METRE. ) );
#12341=ORIENTED_EDGE ( 'NONE', *, *, #16580, .F. ) ;
#12351=CARTESIAN_POINT ( 'NONE',  ( -41.00000000000000711, 53.00000000000000711, -18.00000000000000000 ) ) ;
#12352=VERTEX_POINT ( 'NONE', #14615 ) ;
#12356=EDGE_CURVE ( 'NONE', #16683, #1832, #17278, .T. ) ;
#12357=CARTESIAN_POINT ( 'NONE',  ( -41.00000000000000711, 110.0000000000000000, -19.00000000000000000 ) ) ;
#12363=CYLINDRICAL_SURFACE ( 'NONE', #14283, 2.649999999999992806 ) ;
#12369=CARTESIAN_POINT ( 'NONE',  ( -32.50000000000000000, 53.00000000000000711, -35.00000000000000000 ) ) ;
#12370=ORIENTED_EDGE ( 'NONE', *, *, #17683, .T. ) ;
#12377=VECTOR ( 'NONE', #2651, 1000.000000000000000 ) ;
#12378=CARTESIAN_POINT ( 'NONE',  ( -25.00000000000000000, 110.0000000000000000, 30.00000000000000000 ) ) ;
#12388=CARTESIAN_POINT ( 'NONE',  ( -41.00000000000000711, 110.0000000000000000, 1.500000000000001332 ) ) ;
#12390=AXIS2_PLACEMENT_3D ( 'NONE', #15269, #1838, #7822 ) ;
#12391=ORIENTED_EDGE ( 'NONE', *, *, #18936, .F. ) ;
#12398=VECTOR ( 'NONE', #1734, 1000.000000000000000 ) ;
#12403=VECTOR ( 'NONE', #9635, 1000.000000000000000 ) ;
#12409=LINE ( 'NONE', #361, #2075 ) ;
#12413=AXIS2_PLACEMENT_3D ( 'NONE', #12369, #417, #10992 ) ;
#12419=CARTESIAN_POINT ( 'NONE',  ( -41.00000000000000711, 53.00000000000000711, 26.50000000000000000 ) ) ;
#12423=VERTEX_POINT ( 'NONE', #1385 ) ;
#12433=DIRECTION ( 'NONE',  ( 0.000000000000000000, 0.000000000000000000, 1.000000000000000000 ) ) ;
#12439=ORIENTED_EDGE ( 'NONE', *, *, #3646, .F. ) ;
#12440=ORIENTED_EDGE ( 'NONE', *, *, #866, .T. ) ;
#12445=ORIENTED_EDGE ( 'NONE', *, *, #4554, .T. ) ;
#12447=ORIENTED_EDGE ( 'NONE', *, *, #2832, .T. ) ;
#12453=CARTESIAN_POINT ( 'NONE',  ( -41.00000000000000711, 53.00000000000000711, -38.50000000000000711 ) ) ;
#12457=LINE ( 'NONE', #18454, #14724 ) ;
#12466=EDGE_LOOP ( 'NONE', ( #2959, #10169, #15406, #15981 ) ) ;
#12471=EDGE_CURVE ( 'NONE', #9436, #17811, #11757, .T. ) ;
#12473=VECTOR ( 'NONE', #3489, 1000.000000000000000 ) ;
#12486=EDGE_CURVE ( 'NONE', #5657, #9274, #17857, .T. ) ;
#12489=CARTESIAN_POINT ( 'NONE',  ( -24.00000000000000000, 53.00000000000000711, 27.50000000000000000 ) ) ;
#12500=VECTOR ( 'NONE', #3022, 1000.000000000000000 ) ;
#12518=ORIENTED_EDGE ( 'NONE', *, *, #15123, .F. ) ;
#12531=ORIENTED_EDGE ( 'NONE', *, *, #11906, .F. ) ;
#12537=VERTEX_POINT ( 'NONE', #5116 ) ;
#12540=VECTOR ( 'NONE', #18154, 1000.000000000000000 ) ;
#12546=VECTOR ( 'NONE', #1666, 1000.000000000000000 ) ;
#12549=DIRECTION ( 'NONE',  ( 1.000000000000000000, -0.000000000000000000, -0.000000000000000000 ) ) ;
#12550=ORIENTED_EDGE ( 'NONE', *, *, #7198, .F. ) ;
#12551=CARTESIAN_POINT ( 'NONE',  ( -41.00000000000000711, 110.0000000000000000, -25.50000000000000000 ) ) ;
#12561=VECTOR ( 'NONE', #11469, 1000.000000000000000 ) ;
#12562=PLANE ( 'NONE',  #1467 ) ;
#12568=CARTESIAN_POINT ( 'NONE',  ( -25.00000000000000711, 110.0000000000000000, 0.5000000000000004441 ) ) ;
#12571=VECTOR ( 'NONE', #13895, 1000.000000000000000 ) ;
#12573=LINE ( 'NONE', #5036, #16283 ) ;
#12584=CARTESIAN_POINT ( 'NONE',  ( -41.00000000000000711, 110.0000000000000000, -30.99999999999999645 ) ) ;
#12610=FACE_OUTER_BOUND ( 'NONE', #3306, .T. ) ;
#12613=VERTEX_POINT ( 'NONE', #11071 ) ;
#12622=LINE ( 'NONE', #6463, #12852 ) ;
#12636=VERTEX_POINT ( 'NONE', #588 ) ;
#12644=EDGE_CURVE ( 'NONE', #18999, #6640, #304, .T. ) ;
#12655=CARTESIAN_POINT ( 'NONE',  ( -41.00000000000000711, 53.00000000000000711, -12.50000000000000000 ) ) ;
#12667=LINE ( 'NONE', #6414, #9544 ) ;
#12670=DIRECTION ( 'NONE',  ( 1.000000000000000000, -0.000000000000000000, -0.000000000000000000 ) ) ;
#12671=DIRECTION ( 'NONE',  ( 0.000000000000000000, -1.000000000000000000, 0.000000000000000000 ) ) ;
#12680=PLANE ( 'NONE',  #7824 ) ;
#12684=DIRECTION ( 'NONE',  ( 1.000000000000000000, -0.000000000000000000, -0.000000000000000000 ) ) ;
#12690=LINE ( 'NONE', #6636, #12731 ) ;
#12692=CARTESIAN_POINT ( 'NONE',  ( -41.00000000000000711, 110.0000000000000000, -6.000000000000001776 ) ) ;
#12697=CARTESIAN_POINT ( 'NONE',  ( -41.00000000000000711, 110.0000000000000000, -18.00000000000000000 ) ) ;
#12700=VECTOR ( 'NONE', #3871, 1000.000000000000000 ) ;
#12702=ORIENTED_EDGE ( 'NONE', *, *, #1423, .T. ) ;
#12708=EDGE_CURVE ( 'NONE', #19128, #13505, #2065, .T. ) ;
#12709=PLANE ( 'NONE',  #7546 ) ;
#12715=ORIENTED_EDGE ( 'NONE', *, *, #13297, .F. ) ;
#12717=ORIENTED_EDGE ( 'NONE', *, *, #5642, .T. ) ;
#12725=DIRECTION ( 'NONE',  ( 0.000000000000000000, -1.000000000000000000, -0.000000000000000000 ) ) ;
#12729=DIRECTION ( 'NONE',  ( 0.000000000000000000, -1.000000000000000000, -0.000000000000000000 ) ) ;
#12731=VECTOR ( 'NONE', #14171, 1000.000000000000000 ) ;
#12733=ORIENTED_EDGE ( 'NONE', *, *, #16815, .T. ) ;
#12736=LINE ( 'NONE', #783, #15014 ) ;
#12743=VERTEX_POINT ( 'NONE', #12351 ) ;
#12757=EDGE_CURVE ( 'NONE', #13505, #2590, #9695, .T. ) ;
#12758=LINE ( 'NONE', #19034, #8303 ) ;
#12759=CARTESIAN_POINT ( 'NONE',  ( -24.00000000000000711, 53.00000000000000711, 1.500000000000001332 ) ) ;
#12760=CARTESIAN_POINT ( 'NONE',  ( -40.00000000000000711, 110.0000000000000000, -38.50000000000000711 ) ) ;
#12781=LINE ( 'NONE', #18779, #193 ) ;
#12787=CARTESIAN_POINT ( 'NONE',  ( -41.00000000000000711, 110.0000000000000000, 27.50000000000000000 ) ) ;
#12789=AXIS2_PLACEMENT_3D ( 'NONE', #13106, #14492, #8420 ) ;
#12791=VERTEX_POINT ( 'NONE', #4108 ) ;
#12799=CARTESIAN_POINT ( 'NONE',  ( -41.00000000000000711, 110.0000000000000000, -18.00000000000000000 ) ) ;
#12802=ORIENTED_EDGE ( 'NONE', *, *, #9476, .T. ) ;
#12811=EDGE_CURVE ( 'NONE', #17473, #10091, #17435, .T. ) ;
#12816=ORIENTED_EDGE ( 'NONE', *, *, #2414, .T. ) ;
#12817=ADVANCED_FACE ( 'NONE', ( #870 ), #4005, .T. ) ;
#12820=PLANE ( 'NONE',  #5034 ) ;
#12824=LINE ( 'NONE', #17073, #10943 ) ;
#12836=CARTESIAN_POINT ( 'NONE',  ( -24.00000000000000000, 53.00000000000000711, -32.00000000000000000 ) ) ;
#12844=ORIENTED_EDGE ( 'NONE', *, *, #3873, .T. ) ;
#12845=DIRECTION ( 'NONE',  ( 1.000000000000000000, -0.000000000000000000, -0.000000000000000000 ) ) ;
#12847=VERTEX_POINT ( 'NONE', #6764 ) ;
#12852=VECTOR ( 'NONE', #16959, 1000.000000000000000 ) ;
#12855=ADVANCED_FACE ( 'NONE', ( #11532 ), #12820, .F. ) ;
#12857=EDGE_CURVE ( 'NONE', #19005, #2170, #14212, .T. ) ;
#12860=ORIENTED_EDGE ( 'NONE', *, *, #2677, .T. ) ;
#12863=VECTOR ( 'NONE', #18555, 1000.000000000000000 ) ;
#12869=CARTESIAN_POINT ( 'NONE',  ( -25.00000000000000000, 110.0000000000000000, -11.50000000000000355 ) ) ;
#12877=EDGE_CURVE ( 'NONE', #12352, #16642, #17341, .T. ) ;
#12879=AXIS2_PLACEMENT_3D ( 'NONE', #11764, #18940, #2656 ) ;
#12880=LINE ( 'NONE', #2488, #11790 ) ;
#12882=LINE ( 'NONE', #9929, #11448 ) ;
#12883=CIRCLE ( 'NONE', #5089, 2.649999999999985700 ) ;
#12906=ORIENTED_EDGE ( 'NONE', *, *, #15975, .T. ) ;
#12910=CARTESIAN_POINT ( 'NONE',  ( -41.00000000000000711, 53.00000000000000711, 14.50000000000000000 ) ) ;
#12913=ORIENTED_EDGE ( 'NONE', *, *, #8995, .T. ) ;
#12915=ORIENTED_EDGE ( 'NONE', *, *, #8785, .T. ) ;
#12918=ORIENTED_EDGE ( 'NONE', *, *, #4485, .T. ) ;
#12921=CARTESIAN_POINT ( 'NONE',  ( -24.00000000000000000, 53.00000000000000711, 30.00000000000000000 ) ) ;
#12927=VERTEX_POINT ( 'NONE', #7039 ) ;
#12930=CARTESIAN_POINT ( 'NONE',  ( -40.00000000000000711, 110.0000000000000000, -30.99999999999999645 ) ) ;
#12931=ORIENTED_EDGE ( 'NONE', *, *, #1518, .F. ) ;
#12934=ORIENTED_EDGE ( 'NONE', *, *, #15152, .T. ) ;
#12940=PLANE ( 'NONE',  #11247 ) ;
#12945=VECTOR ( 'NONE', #9156, 1000.000000000000000 ) ;
#12963=CARTESIAN_POINT ( 'NONE',  ( -41.00000000000000711, 113.0000000000000000, 30.00000000000000000 ) ) ;
#12965=CARTESIAN_POINT ( 'NONE',  ( -25.00000000000000711, 110.0000000000000000, -38.50000000000000711 ) ) ;
#12966=LINE ( 'NONE', #17389, #649 ) ;
#12973=VERTEX_POINT ( 'NONE', #7606 ) ;
#12988=LINE ( 'NONE', #2605, #2073 ) ;
#12989=VERTEX_POINT ( 'NONE', #10625 ) ;
#12993=ORIENTED_EDGE ( 'NONE', *, *, #17683, .F. ) ;
#12996=ORIENTED_EDGE ( 'NONE', *, *, #15511, .F. ) ;
#12997=PRODUCT ( 'Heating Element & carriage', 'Heating Element & carriage', '', ( #15 ) ) ;
#13007=DIRECTION ( 'NONE',  ( -0.000000000000000000, -0.000000000000000000, -1.000000000000000000 ) ) ;
#13008=ORIENTED_EDGE ( 'NONE', *, *, #17300, .T. ) ;
#13012=DIRECTION ( 'NONE',  ( 0.000000000000000000, 0.000000000000000000, 1.000000000000000000 ) ) ;
#13021=VERTEX_POINT ( 'NONE', #14589 ) ;
#13026=AXIS2_PLACEMENT_3D ( 'NONE', #7078, #16009, #5331 ) ;
#13040=FACE_BOUND ( 'NONE', #2632, .T. ) ;
#13054=EDGE_CURVE ( 'NONE', #10947, #7234, #249, .T. ) ;
#13062=EDGE_CURVE ( 'NONE', #15286, #19005, #10067, .T. ) ;
#13065=LINE ( 'NONE', #19061, #18676 ) ;
#13067=EDGE_CURVE ( 'NONE', #1273, #3857, #18201, .T. ) ;
#13070=FACE_OUTER_BOUND ( 'NONE', #10475, .T. ) ;
#13078=CARTESIAN_POINT ( 'NONE',  ( -25.00000000000000000, 110.0000000000000000, -44.00000000000000000 ) ) ;
#13088=EDGE_CURVE ( 'NONE', #19248, #2931, #13771, .T. ) ;
#13091=ORIENTED_EDGE ( 'NONE', *, *, #3396, .F. ) ;
#13100=LINE ( 'NONE', #5669, #3133 ) ;
#13103=ORIENTED_EDGE ( 'NONE', *, *, #6149, .F. ) ;
#13106=CARTESIAN_POINT ( 'NONE',  ( -41.00000000000000711, 110.0000000000000000, -11.50000000000000000 ) ) ;
#13108=VECTOR ( 'NONE', #7306, 1000.000000000000000 ) ;
#13111=CARTESIAN_POINT ( 'NONE',  ( -32.50000000000000000, 52.00000000000000711, 15.00000000000000000 ) ) ;
#13114=CIRCLE ( 'NONE', #4378, 2.649999999999999467 ) ;
#13117=ORIENTED_EDGE ( 'NONE', *, *, #5296, .F. ) ;
#13118=ORIENTED_EDGE ( 'NONE', *, *, #16957, .T. ) ;
#13120=FACE_OUTER_BOUND ( 'NONE', #3949, .T. ) ;
#13124=LINE ( 'NONE', #1282, #1236 ) ;
#13126=ORIENTED_EDGE ( 'NONE', *, *, #11034, .T. ) ;
#13130=VERTEX_POINT ( 'NONE', #12000 ) ;
#13132=ORIENTED_EDGE ( 'NONE', *, *, #1619, .T. ) ;
#13139=DIRECTION ( 'NONE',  ( -0.000000000000000000, 1.000000000000000000, -0.000000000000000000 ) ) ;
#13153=DIRECTION ( 'NONE',  ( 1.000000000000000000, 0.000000000000000000, 0.000000000000000000 ) ) ;
#13156=DIRECTION ( 'NONE',  ( 1.000000000000000000, -0.000000000000000000, -0.000000000000000000 ) ) ;
#13165=VECTOR ( 'NONE', #1058, 1000.000000000000000 ) ;
#13169=DIRECTION ( 'NONE',  ( 0.000000000000000000, 0.000000000000000000, -1.000000000000000000 ) ) ;
#13185=DIRECTION ( 'NONE',  ( 0.000000000000000000, 0.000000000000000000, -1.000000000000000000 ) ) ;
#13190=EDGE_CURVE ( 'NONE', #1572, #1380, #15344, .T. ) ;
#13197=ORIENTED_EDGE ( 'NONE', *, *, #8903, .T. ) ;
#13227=EDGE_LOOP ( 'NONE', ( #16602, #10456, #8783, #17559 ) ) ;
#13229=DIRECTION ( 'NONE',  ( -1.156482317317871478E-16, 1.000000000000000000, 0.000000000000000000 ) ) ;
#13236=LINE ( 'NONE', #5799, #5367 ) ;
#13240=CARTESIAN_POINT ( 'NONE',  ( -24.00000000000000711, 53.00000000000000711, 0.5000000000000004441 ) ) ;
#13256=CARTESIAN_POINT ( 'NONE',  ( -32.50000000000000000, 52.00000000000000711, 17.64999999999999858 ) ) ;
#13262=CARTESIAN_POINT ( 'NONE',  ( -41.00000000000000711, 53.00000000000000711, -25.50000000000000000 ) ) ;
#13278=LINE ( 'NONE', #11811, #14609 ) ;
#13280=CARTESIAN_POINT ( 'NONE',  ( -41.00000000000000711, 53.00000000000000711, 14.50000000000000000 ) ) ;
#13282=VERTEX_POINT ( 'NONE', #733 ) ;
#13285=DIRECTION ( 'NONE',  ( 1.000000000000000000, -0.000000000000000000, -0.000000000000000000 ) ) ;
#13295=ORIENTED_EDGE ( 'NONE', *, *, #19263, .F. ) ;
#13297=EDGE_CURVE ( 'NONE', #3528, #4404, #2204, .T. ) ;
#13299=CARTESIAN_POINT ( 'NONE',  ( -25.00000000000000000, 110.0000000000000000, 30.00000000000000000 ) ) ;
#13300=LINE ( 'NONE', #18124, #5108 ) ;
#13303=LINE ( 'NONE', #10462, #15334 ) ;
#13304=ADVANCED_FACE ( 'NONE', ( #11202 ), #17021, .T. ) ;
#13307=AXIS2_PLACEMENT_3D ( 'NONE', #14030, #12272, #4739 ) ;
#13314=CARTESIAN_POINT ( 'NONE',  ( -40.00000000000000711, 110.0000000000000000, 30.00000000000000000 ) ) ;
#13327=AXIS2_PLACEMENT_3D ( 'NONE', #11009, #6885, #14051 ) ;
#13331=EDGE_CURVE ( 'NONE', #3796, #4121, #916, .T. ) ;
#13332=CARTESIAN_POINT ( 'NONE',  ( -25.00000000000000711, 53.00000000000000711, -6.000000000000001776 ) ) ;
#13334=DIRECTION ( 'NONE',  ( 0.000000000000000000, 0.000000000000000000, 1.000000000000000000 ) ) ;
#13338=CARTESIAN_POINT ( 'NONE',  ( -25.00000000000000000, 53.00000000000000711, 21.00000000000000000 ) ) ;
#13376=LINE ( 'NONE', #17698, #6600 ) ;
#13381=DIRECTION ( 'NONE',  ( 0.000000000000000000, 0.000000000000000000, -1.000000000000000000 ) ) ;
#13387=CARTESIAN_POINT ( 'NONE',  ( -41.00000000000000711, 53.00000000000000711, 13.50000000000000000 ) ) ;
#13388=VERTEX_POINT ( 'NONE', #4254 ) ;
#13397=VECTOR ( 'NONE', #1727, 1000.000000000000000 ) ;
#13406=ORIENTED_EDGE ( 'NONE', *, *, #2246, .F. ) ;
#13417=DIRECTION ( 'NONE',  ( 0.000000000000000000, 0.000000000000000000, -1.000000000000000000 ) ) ;
#13426=ORIENTED_EDGE ( 'NONE', *, *, #18361, .T. ) ;
#13427=DIRECTION ( 'NONE',  ( -1.156482317317871478E-16, 1.000000000000000000, 0.000000000000000000 ) ) ;
#13434=DIRECTION ( 'NONE',  ( -1.000000000000000000, 0.000000000000000000, -0.000000000000000000 ) ) ;
#13435=EDGE_CURVE ( 'NONE', #16948, #10054, #8560, .T. ) ;
#13459=EDGE_CURVE ( 'NONE', #1673, #9439, #11684, .T. ) ;
#13462=DIRECTION ( 'NONE',  ( 0.000000000000000000, -0.000000000000000000, 1.000000000000000000 ) ) ;
#13473=VECTOR ( 'NONE', #9516, 1000.000000000000000 ) ;
#13477=ADVANCED_FACE ( 'NONE', ( #4161 ), #10112, .F. ) ;
#13482=CARTESIAN_POINT ( 'NONE',  ( -41.00000000000000711, 53.00000000000000711, 20.00000000000000000 ) ) ;
#13487=CARTESIAN_POINT ( 'NONE',  ( -25.00000000000000000, 53.00000000000000711, 30.00000000000000000 ) ) ;
#13489=LINE ( 'NONE', #11010, #7390 ) ;
#13494=ORIENTED_EDGE ( 'NONE', *, *, #14904, .F. ) ;
#13500=AXIS2_PLACEMENT_3D ( 'NONE', #19179, #4382, #17806 ) ;
#13505=VERTEX_POINT ( 'NONE', #234 ) ;
#13511=CARTESIAN_POINT ( 'NONE',  ( -41.00000000000000711, 53.00000000000000711, 8.000000000000000000 ) ) ;
#13514=VECTOR ( 'NONE', #7665, 1000.000000000000000 ) ;
#13521=PLANE ( 'NONE',  #17124 ) ;
#13525=EDGE_CURVE ( 'NONE', #2239, #6673, #3173, .T. ) ;
#13527=DIRECTION ( 'NONE',  ( -0.000000000000000000, 1.000000000000000000, -0.000000000000000000 ) ) ;
#13531=CARTESIAN_POINT ( 'NONE',  ( -40.00000000000000711, 110.0000000000000000, 6.999999999999999112 ) ) ;
#13535=LINE ( 'NONE', #16876, #12540 ) ;
#13539=CARTESIAN_POINT ( 'NONE',  ( -41.00000000000000711, 53.00000000000000711, -12.50000000000000000 ) ) ;
#13541=LINE ( 'NONE', #13338, #16461 ) ;
#13556=DIRECTION ( 'NONE',  ( -1.156482317317871478E-16, 1.000000000000000000, 0.000000000000000000 ) ) ;
#13569=CARTESIAN_POINT ( 'NONE',  ( -24.00000000000000000, 110.0000000000000000, 30.00000000000000000 ) ) ;
#13577=LINE ( 'NONE', #16528, #5070 ) ;
#13588=EDGE_LOOP ( 'NONE', ( #11979, #8816, #10585, #13126 ) ) ;
#13589=ORIENTED_EDGE ( 'NONE', *, *, #11976, .T. ) ;
#13596=ORIENTED_EDGE ( 'NONE', *, *, #11069, .F. ) ;
#13602=VERTEX_POINT ( 'NONE', #7385 ) ;
#13606=CARTESIAN_POINT ( 'NONE',  ( -41.00000000000000711, 110.0000000000000000, 1.500000000000001332 ) ) ;
#13608=ADVANCED_FACE ( 'NONE', ( #6118 ), #18081, .T. ) ;
#13609=ORIENTED_EDGE ( 'NONE', *, *, #6149, .T. ) ;
#13625=EDGE_LOOP ( 'NONE', ( #13903, #804, #17839, #15656 ) ) ;
#13632=AXIS2_PLACEMENT_3D ( 'NONE', #3205, #8013, #4789 ) ;
#13633=FACE_OUTER_BOUND ( 'NONE', #14509, .T. ) ;
#13634=DIRECTION ( 'NONE',  ( -0.000000000000000000, 1.000000000000000000, -0.000000000000000000 ) ) ;
#13646=VERTEX_POINT ( 'NONE', #14940 ) ;
#13657=CARTESIAN_POINT ( 'NONE',  ( -24.00000000000000711, 53.00000000000000711, 20.00000000000000000 ) ) ;
#13666=MECHANICAL_DESIGN_GEOMETRIC_PRESENTATION_REPRESENTATION('',(#6795),#5542);
#13675=CARTESIAN_POINT ( 'NONE',  ( -40.00000000000000711, 53.00000000000000711, 1.500000000000001332 ) ) ;
#13680=DIRECTION ( 'NONE',  ( -0.000000000000000000, -0.000000000000000000, -1.000000000000000000 ) ) ;
#13688=ORIENTED_EDGE ( 'NONE', *, *, #7602, .F. ) ;
#13695=ORIENTED_EDGE ( 'NONE', *, *, #4751, .T. ) ;
#13697=EDGE_LOOP ( 'NONE', ( #8130, #3626, #17241, #11370 ) ) ;
#13701=CARTESIAN_POINT ( 'NONE',  ( -25.00000000000000000, 53.00000000000000711, 30.00000000000000000 ) ) ;
#13706=EDGE_CURVE ( 'NONE', #11249, #13021, #3752, .T. ) ;
#13710=ORIENTED_EDGE ( 'NONE', *, *, #7719, .F. ) ;
#13713=CARTESIAN_POINT ( 'NONE',  ( 0.000000000000000000, 0.000000000000000000, 0.000000000000000000 ) ) ;
#13729=FACE_BOUND ( 'NONE', #1728, .T. ) ;
#13731=CARTESIAN_POINT ( 'NONE',  ( -40.00000000000000000, 53.00000000000000711, -50.00000000000000000 ) ) ;
#13747=ORIENTED_EDGE ( 'NONE', *, *, #6126, .F. ) ;
#13752=CARTESIAN_POINT ( 'NONE',  ( -41.00000000000000711, 53.00000000000000711, -12.50000000000000000 ) ) ;
#13756=LINE ( 'NONE', #1094, #11698 ) ;
#13769=PLANE ( 'NONE',  #12283 ) ;
#13771=LINE ( 'NONE', #16060, #6102 ) ;
#13773=VECTOR ( 'NONE', #12549, 1000.000000000000000 ) ;
#13778=CARTESIAN_POINT ( 'NONE',  ( -41.00000000000000711, 110.0000000000000000, 6.999999999999999112 ) ) ;
#13779=VECTOR ( 'NONE', #14232, 1000.000000000000000 ) ;
#13788=ORIENTED_EDGE ( 'NONE', *, *, #8811, .T. ) ;
#13799=AXIS2_PLACEMENT_3D ( 'NONE', #17560, #17957, #4529 ) ;
#13803=EDGE_CURVE ( 'NONE', #6518, #17050, #12667, .T. ) ;
#13810=ORIENTED_EDGE ( 'NONE', *, *, #12249, .F. ) ;
#13814=VERTEX_POINT ( 'NONE', #11097 ) ;
#13829=EDGE_LOOP ( 'NONE', ( #9230, #11424, #16656, #2527 ) ) ;
#13832=CARTESIAN_POINT ( 'NONE',  ( -25.00000000000000711, 110.0000000000000000, 26.50000000000000000 ) ) ;
#13834=DIRECTION ( 'NONE',  ( -0.000000000000000000, -0.000000000000000000, -1.000000000000000000 ) ) ;
#13838=LINE ( 'NONE', #506, #16288 ) ;
#13839=VECTOR ( 'NONE', #14677, 1000.000000000000000 ) ;
#13842=ORIENTED_EDGE ( 'NONE', *, *, #16957, .F. ) ;
#13844=DIRECTION ( 'NONE',  ( 1.000000000000000000, -0.000000000000000000, -0.000000000000000000 ) ) ;
#13858=DIRECTION ( 'NONE',  ( 1.000000000000000000, 0.000000000000000000, 0.000000000000000000 ) ) ;
#13859=DIRECTION ( 'NONE',  ( 1.000000000000000000, -0.000000000000000000, -0.000000000000000000 ) ) ;
#13861=DIRECTION ( 'NONE',  ( -1.000000000000000000, 0.000000000000000000, -0.000000000000000000 ) ) ;
#13862=ADVANCED_FACE ( 'NONE', ( #2184 ), #9442, .T. ) ;
#13863=ORIENTED_EDGE ( 'NONE', *, *, #2398, .F. ) ;
#13869=EDGE_CURVE ( 'NONE', #13949, #14586, #7784, .T. ) ;
#13876=CARTESIAN_POINT ( 'NONE',  ( -24.00000000000000000, 53.00000000000000711, 30.00000000000000000 ) ) ;
#13880=DIRECTION ( 'NONE',  ( 1.000000000000000000, -0.000000000000000000, -0.000000000000000000 ) ) ;
#13892=ORIENTED_EDGE ( 'NONE', *, *, #1384, .T. ) ;
#13893=EDGE_LOOP ( 'NONE', ( #5490, #3140, #3235, #16374 ) ) ;
#13895=DIRECTION ( 'NONE',  ( -1.156482317317871478E-16, 1.000000000000000000, 0.000000000000000000 ) ) ;
#13898=CARTESIAN_POINT ( 'NONE',  ( -24.00000000000000000, 110.0000000000000000, -38.50000000000000711 ) ) ;
#13902=VERTEX_POINT ( 'NONE', #430 ) ;
#13903=ORIENTED_EDGE ( 'NONE', *, *, #15975, .F. ) ;
#13911=EDGE_CURVE ( 'NONE', #5613, #1200, #12758, .T. ) ;
#13917=EDGE_CURVE ( 'NONE', #2170, #5957, #17366, .T. ) ;
#13918=LINE ( 'NONE', #12258, #10663 ) ;
#13922=CARTESIAN_POINT ( 'NONE',  ( -25.00000000000000711, 110.0000000000000000, -32.00000000000000000 ) ) ;
#13925=DIRECTION ( 'NONE',  ( 0.000000000000000000, -0.000000000000000000, 1.000000000000000000 ) ) ;
#13926=EDGE_CURVE ( 'NONE', #4628, #6193, #17561, .T. ) ;
#13927=CARTESIAN_POINT ( 'NONE',  ( -41.00000000000000711, 110.0000000000000000, 21.00000000000000000 ) ) ;
#13936=ORIENTED_EDGE ( 'NONE', *, *, #15140, .F. ) ;
#13947=VECTOR ( 'NONE', #409, 1000.000000000000000 ) ;
#13949=VERTEX_POINT ( 'NONE', #16086 ) ;
#13956=CARTESIAN_POINT ( 'NONE',  ( -24.00000000000000711, 53.00000000000000711, -32.00000000000000000 ) ) ;
#13957=DIRECTION ( 'NONE',  ( 0.000000000000000000, -1.000000000000000000, -0.000000000000000000 ) ) ;
#13959=VECTOR ( 'NONE', #5685, 1000.000000000000000 ) ;
#13960=EDGE_LOOP ( 'NONE', ( #4528, #9203, #16277, #15479, #18992, #15884, #12224, #6678, #2919, #15755, #9047, #11520, #4813, #6816, #9948, #12844, #12550, #6606, #2132, #9148, #18069, #15956, #18863, #13008, #11412, #15862, #12913, #8500, #10773, #1659, #13788, #7422, #17068, #8134, #4712, #10227, #7040, #4795, #18633, #2449, #14475, #10993, #19301, #17547, #7417, #11627, #13892, #8980, #10484, #5475, #12325, #8607 ) ) ;
#13965=CARTESIAN_POINT ( 'NONE',  ( -25.00000000000000000, 53.00000000000000711, -38.50000000000000711 ) ) ;
#13976=CARTESIAN_POINT ( 'NONE',  ( -41.00000000000000711, 53.00000000000000711, -11.50000000000000000 ) ) ;
#13981=ORIENTED_EDGE ( 'NONE', *, *, #7485, .T. ) ;
#13993=EDGE_LOOP ( 'NONE', ( #10145, #19288 ) ) ;
#14005=VERTEX_POINT ( 'NONE', #17656 ) ;
#14007=ORIENTED_EDGE ( 'NONE', *, *, #16721, .T. ) ;
#14022=FACE_BOUND ( 'NONE', #343, .T. ) ;
#14030=CARTESIAN_POINT ( 'NONE',  ( -41.00000000000000711, 110.0000000000000000, 14.50000000000000000 ) ) ;
#14041=LINE ( 'NONE', #3559, #1228 ) ;
#14050=LINE ( 'NONE', #9447, #4105 ) ;
#14051=DIRECTION ( 'NONE',  ( -1.000000000000000000, 0.000000000000000000, -0.000000000000000000 ) ) ;
#14067=CARTESIAN_POINT ( 'NONE',  ( -41.00000000000000711, 53.00000000000000711, -18.00000000000000000 ) ) ;
#14071=VECTOR ( 'NONE', #995, 1000.000000000000000 ) ;
#14076=LINE ( 'NONE', #14173, #16795 ) ;
#14085=CARTESIAN_POINT ( 'NONE',  ( -41.00000000000000711, 53.00000000000000711, -11.50000000000000000 ) ) ;
#14091=CARTESIAN_POINT ( 'NONE',  ( -41.00000000000000711, 110.0000000000000000, -44.00000000000000000 ) ) ;
#14102=ORIENTED_EDGE ( 'NONE', *, *, #17086, .T. ) ;
#14105=VECTOR ( 'NONE', #3955, 1000.000000000000000 ) ;
#14124=DIRECTION ( 'NONE',  ( 0.000000000000000000, -1.000000000000000000, -0.000000000000000000 ) ) ;
#14129=VECTOR ( 'NONE', #18574, 1000.000000000000000 ) ;
#14132=ORIENTED_EDGE ( 'NONE', *, *, #6997, .T. ) ;
#14138=CARTESIAN_POINT ( 'NONE',  ( -25.00000000000000000, 53.00000000000000711, 26.50000000000000000 ) ) ;
#14141=ORIENTED_EDGE ( 'NONE', *, *, #15282, .T. ) ;
#14142=VECTOR ( 'NONE', #358, 1000.000000000000000 ) ;
#14146=DIRECTION ( 'NONE',  ( -1.000000000000000000, 0.000000000000000000, -0.000000000000000000 ) ) ;
#14150=DIRECTION ( 'NONE',  ( 0.000000000000000000, -1.000000000000000000, 0.000000000000000000 ) ) ;
#14152=PLANE ( 'NONE',  #13327 ) ;
#14153=LINE ( 'NONE', #16532, #18965 ) ;
#14171=DIRECTION ( 'NONE',  ( 0.000000000000000000, 0.000000000000000000, -1.000000000000000000 ) ) ;
#14173=CARTESIAN_POINT ( 'NONE',  ( -41.00000000000000711, 53.00000000000000711, 1.500000000000001332 ) ) ;
#14176=ORIENTED_EDGE ( 'NONE', *, *, #3157, .F. ) ;
#14178=EDGE_CURVE ( 'NONE', #9439, #19394, #10489, .T. ) ;
#14185=ORIENTED_EDGE ( 'NONE', *, *, #7349, .F. ) ;
#14192=DIRECTION ( 'NONE',  ( 0.000000000000000000, -1.000000000000000000, 0.000000000000000000 ) ) ;
#14194=LINE ( 'NONE', #10049, #14272 ) ;
#14210=LINE ( 'NONE', #8604, #13165 ) ;
#14212=LINE ( 'NONE', #8245, #17854 ) ;
#14220=LINE ( 'NONE', #8155, #15053 ) ;
#14230=CARTESIAN_POINT ( 'NONE',  ( -41.00000000000000711, 110.0000000000000000, -45.00000000000000000 ) ) ;
#14232=DIRECTION ( 'NONE',  ( 1.000000000000000000, -0.000000000000000000, -0.000000000000000000 ) ) ;
#14233=ORIENTED_EDGE ( 'NONE', *, *, #7832, .T. ) ;
#14235=ORIENTED_EDGE ( 'NONE', *, *, #11623, .T. ) ;
#14272=VECTOR ( 'NONE', #17809, 1000.000000000000000 ) ;
#14275=EDGE_LOOP ( 'NONE', ( #6377, #11402, #2423, #17582 ) ) ;
#14276=DIRECTION ( 'NONE',  ( -1.156482317317871478E-16, 1.000000000000000000, 0.000000000000000000 ) ) ;
#14278=DIRECTION ( 'NONE',  ( 1.000000000000000000, -0.000000000000000000, -0.000000000000000000 ) ) ;
#14283=AXIS2_PLACEMENT_3D ( 'NONE', #7967, #11260, #2168 ) ;
#14288=( LENGTH_UNIT ( ) NAMED_UNIT ( * ) SI_UNIT ( .MILLI., .METRE. ) );
#14291=ORIENTED_EDGE ( 'NONE', *, *, #11675, .T. ) ;
#14297=VERTEX_POINT ( 'NONE', #15500 ) ;
#14299=CARTESIAN_POINT ( 'NONE',  ( -24.00000000000000711, 53.00000000000000711, -45.00000000000000000 ) ) ;
#14300=EDGE_LOOP ( 'NONE', ( #15770, #18334, #19153, #4599 ) ) ;
#14302=EDGE_CURVE ( 'NONE', #3842, #853, #309, .T. ) ;
#14303=DIRECTION ( 'NONE',  ( -1.000000000000000000, 0.000000000000000000, -0.000000000000000000 ) ) ;
#14307=PLANE ( 'NONE',  #9376 ) ;
#14312=DIRECTION ( 'NONE',  ( -1.000000000000000000, 0.000000000000000000, -0.000000000000000000 ) ) ;
#14321=EDGE_CURVE ( 'NONE', #6553, #16539, #16984, .T. ) ;
#14324=DIRECTION ( 'NONE',  ( -1.000000000000000000, 0.000000000000000000, -0.000000000000000000 ) ) ;
#14328=DIRECTION ( 'NONE',  ( -1.000000000000000000, 0.000000000000000000, -0.000000000000000000 ) ) ;
#14330=DIRECTION ( 'NONE',  ( 1.000000000000000000, -0.000000000000000000, -0.000000000000000000 ) ) ;
#14331=SURFACE_STYLE_FILL_AREA ( #2285 ) ;
#14335=ORIENTED_EDGE ( 'NONE', *, *, #436, .T. ) ;
#14337=EDGE_CURVE ( 'NONE', #13388, #1370, #3354, .T. ) ;
#14342=LINE ( 'NONE', #7182, #2486 ) ;
#14350=DIRECTION ( 'NONE',  ( 0.000000000000000000, -1.000000000000000000, 0.000000000000000000 ) ) ;
#14355=ADVANCED_FACE ( 'NONE', ( #501, #12265, #5020, #1880, #6489, #9512, #14022, #593, #5123, #11076, #13729, #10688, #15213 ), #7764, .F. ) ;
#14356=CARTESIAN_POINT ( 'NONE',  ( -24.00000000000000000, 53.00000000000000711, 6.999999999999999112 ) ) ;
#14365=DIRECTION ( 'NONE',  ( -0.000000000000000000, -0.000000000000000000, -1.000000000000000000 ) ) ;
#14366=CARTESIAN_POINT ( 'NONE',  ( -41.00000000000000711, 110.0000000000000000, 26.50000000000000000 ) ) ;
#14373=ORIENTED_EDGE ( 'NONE', *, *, #14871, .F. ) ;
#14390=CARTESIAN_POINT ( 'NONE',  ( -41.00000000000000711, 53.00000000000000711, 13.50000000000000000 ) ) ;
#14391=EDGE_LOOP ( 'NONE', ( #4681, #1547, #857, #13842 ) ) ;
#14401=DIRECTION ( 'NONE',  ( 0.000000000000000000, 0.000000000000000000, -1.000000000000000000 ) ) ;
#14402=VECTOR ( 'NONE', #17472, 1000.000000000000000 ) ;
#14408=AXIS2_PLACEMENT_3D ( 'NONE', #15235, #4461, #10609 ) ;
#14413=VECTOR ( 'NONE', #12269, 1000.000000000000000 ) ;
#14415=VERTEX_POINT ( 'NONE', #176 ) ;
#14417=FACE_OUTER_BOUND ( 'NONE', #10279, .T. ) ;
#14420=CARTESIAN_POINT ( 'NONE',  ( -41.00000000000000711, 53.00000000000000711, -32.00000000000000000 ) ) ;
#14423=LINE ( 'NONE', #2460, #3756 ) ;
#14429=FACE_BOUND ( 'NONE', #1247, .T. ) ;
#14433=EDGE_CURVE ( 'NONE', #2609, #5613, #16443, .T. ) ;
#14442=LINE ( 'NONE', #4159, #5021 ) ;
#14450=CARTESIAN_POINT ( 'NONE',  ( -41.00000000000000711, 110.0000000000000000, 8.000000000000000000 ) ) ;
#14470=CARTESIAN_POINT ( 'NONE',  ( -41.00000000000000711, 53.00000000000000711, 20.00000000000000000 ) ) ;
#14474=ORIENTED_EDGE ( 'NONE', *, *, #9455, .F. ) ;
#14475=ORIENTED_EDGE ( 'NONE', *, *, #3944, .F. ) ;
#14483=LINE ( 'NONE', #1054, #13839 ) ;
#14486=ORIENTED_EDGE ( 'NONE', *, *, #10536, .F. ) ;
#14489=CARTESIAN_POINT ( 'NONE',  ( -40.00000000000000000, 53.00000000000000711, 30.00000000000000000 ) ) ;
#14491=LINE ( 'NONE', #14684, #11004 ) ;
#14492=DIRECTION ( 'NONE',  ( 0.000000000000000000, -1.000000000000000000, -0.000000000000000000 ) ) ;
#14497=CARTESIAN_POINT ( 'NONE',  ( -25.00000000000000000, 110.0000000000000000, -37.50000000000000711 ) ) ;
#14501=EDGE_CURVE ( 'NONE', #7135, #4224, #1653, .T. ) ;
#14509=EDGE_LOOP ( 'NONE', ( #6935, #4920, #12033, #3907 ) ) ;
#14515=ORIENTED_EDGE ( 'NONE', *, *, #2222, .F. ) ;
#14525=FACE_OUTER_BOUND ( 'NONE', #8077, .T. ) ;
#14535=VECTOR ( 'NONE', #4778, 1000.000000000000000 ) ;
#14542=EDGE_CURVE ( 'NONE', #18278, #4488, #4396, .T. ) ;
#14549=LINE ( 'NONE', #1418, #10830 ) ;
#14558=EDGE_CURVE ( 'NONE', #4945, #7898, #8112, .T. ) ;
#14569=DIRECTION ( 'NONE',  ( 0.000000000000000000, 0.000000000000000000, -1.000000000000000000 ) ) ;
#14578=ORIENTED_EDGE ( 'NONE', *, *, #16558, .F. ) ;
#14585=ADVANCED_FACE ( 'NONE', ( #12610 ), #6358, .T. ) ;
#14586=VERTEX_POINT ( 'NONE', #3404 ) ;
#14589=CARTESIAN_POINT ( 'NONE',  ( -41.00000000000000711, 110.0000000000000000, 14.50000000000000000 ) ) ;
#14592=LINE ( 'NONE', #12921, #7484 ) ;
#14594=VECTOR ( 'NONE', #17966, 1000.000000000000000 ) ;
#14600=CARTESIAN_POINT ( 'NONE',  ( -40.00000000000000000, 53.00000000000000711, 30.00000000000000000 ) ) ;
#14601=EDGE_LOOP ( 'NONE', ( #1290, #9666, #4988, #15687 ) ) ;
#14606=ORIENTED_EDGE ( 'NONE', *, *, #3873, .F. ) ;
#14609=VECTOR ( 'NONE', #13381, 1000.000000000000000 ) ;
#14615=CARTESIAN_POINT ( 'NONE',  ( -25.00000000000000711, 110.0000000000000000, -25.50000000000000000 ) ) ;
#14619=DIRECTION ( 'NONE',  ( 0.000000000000000000, -1.000000000000000000, 0.000000000000000000 ) ) ;
#14642=DIRECTION ( 'NONE',  ( 1.000000000000000000, -0.000000000000000000, -0.000000000000000000 ) ) ;
#14652=EDGE_CURVE ( 'NONE', #18273, #3614, #9283, .T. ) ;
#14661=CARTESIAN_POINT ( 'NONE',  ( -41.00000000000000711, 53.00000000000000711, 26.50000000000000000 ) ) ;
#14665=ADVANCED_FACE ( 'NONE', ( #658 ), #18417, .T. ) ;
#14666=ORIENTED_EDGE ( 'NONE', *, *, #5296, .T. ) ;
#14667=EDGE_LOOP ( 'NONE', ( #11196, #4976, #11164, #9788 ) ) ;
#14672=VERTEX_POINT ( 'NONE', #12419 ) ;
#14677=DIRECTION ( 'NONE',  ( 0.000000000000000000, 0.000000000000000000, 1.000000000000000000 ) ) ;
#14684=CARTESIAN_POINT ( 'NONE',  ( -25.00000000000000000, 53.00000000000000711, 20.00000000000000000 ) ) ;
#14691=DIRECTION ( 'NONE',  ( 0.000000000000000000, 0.000000000000000000, 1.000000000000000000 ) ) ;
#14694=EDGE_CURVE ( 'NONE', #9587, #7631, #18317, .T. ) ;
#14701=VERTEX_POINT ( 'NONE', #18604 ) ;
#14710=VERTEX_POINT ( 'NONE', #16842 ) ;
#14713=CARTESIAN_POINT ( 'NONE',  ( -40.00000000000000711, 110.0000000000000000, 26.50000000000000000 ) ) ;
#14722=ADVANCED_FACE ( 'NONE', ( #9661 ), #11130, .F. ) ;
#14724=VECTOR ( 'NONE', #3548, 1000.000000000000000 ) ;
#14726=EDGE_LOOP ( 'NONE', ( #8320, #13609, #9990, #6469 ) ) ;
#14735=CARTESIAN_POINT ( 'NONE',  ( -40.00000000000000000, 53.00000000000000711, 30.00000000000000000 ) ) ;
#14740=DIRECTION ( 'NONE',  ( -1.000000000000000000, 0.000000000000000000, -0.000000000000000000 ) ) ;
#14744=VECTOR ( 'NONE', #11852, 1000.000000000000000 ) ;
#14746=CARTESIAN_POINT ( 'NONE',  ( -41.00000000000000711, 110.0000000000000000, -44.00000000000000000 ) ) ;
#14763=FACE_OUTER_BOUND ( 'NONE', #1958, .T. ) ;
#14764=CIRCLE ( 'NONE', #1623, 2.649999999999999467 ) ;
#14768=FACE_OUTER_BOUND ( 'NONE', #8535, .T. ) ;
#14769=EDGE_CURVE ( 'NONE', #12144, #17252, #6857, .T. ) ;
#14772=EDGE_CURVE ( 'NONE', #18998, #1273, #19208, .T. ) ;
#14798=EDGE_CURVE ( 'NONE', #12337, #7234, #15881, .T. ) ;
#14799=PLANE ( 'NONE',  #16624 ) ;
#14803=ORIENTED_EDGE ( 'NONE', *, *, #12757, .F. ) ;
#14819=DIRECTION ( 'NONE',  ( 0.000000000000000000, -1.000000000000000000, 0.000000000000000000 ) ) ;
#14821=CARTESIAN_POINT ( 'NONE',  ( -41.00000000000000711, 53.00000000000000711, -18.00000000000000000 ) ) ;
#14825=( NAMED_UNIT ( * ) PLANE_ANGLE_UNIT ( ) SI_UNIT ( $, .RADIAN. ) );
#14834=ORIENTED_EDGE ( 'NONE', *, *, #18058, .T. ) ;
#14850=STYLED_ITEM ( 'NONE', ( #5422 ), #17097 ) ;
#14858=CARTESIAN_POINT ( 'NONE',  ( -41.00000000000000711, 53.00000000000000711, -11.50000000000000000 ) ) ;
#14861=EDGE_CURVE ( 'NONE', #10054, #11529, #15789, .T. ) ;
#14863=VECTOR ( 'NONE', #6628, 1000.000000000000000 ) ;
#14866=ADVANCED_FACE ( 'NONE', ( #2540 ), #17538, .F. ) ;
#14869=ORIENTED_EDGE ( 'NONE', *, *, #8435, .F. ) ;
#14871=EDGE_CURVE ( 'NONE', #9436, #3842, #11542, .T. ) ;
#14875=VERTEX_POINT ( 'NONE', #17635 ) ;
#14892=DIRECTION ( 'NONE',  ( -1.000000000000000000, 0.000000000000000000, -0.000000000000000000 ) ) ;
#14894=AXIS2_PLACEMENT_3D ( 'NONE', #8523, #2356, #14312 ) ;
#14895=CARTESIAN_POINT ( 'NONE',  ( -24.00000000000000711, 110.0000000000000000, -5.000000000000000888 ) ) ;
#14897=ORIENTED_EDGE ( 'NONE', *, *, #2994, .T. ) ;
#14898=EDGE_LOOP ( 'NONE', ( #14007, #5087, #12993, #12816 ) ) ;
#14902=VERTEX_POINT ( 'NONE', #15067 ) ;
#14904=EDGE_CURVE ( 'NONE', #13602, #209, #15454, .T. ) ;
#14905=EDGE_CURVE ( 'NONE', #1350, #7469, #10540, .T. ) ;
#14912=LINE ( 'NONE', #18347, #11293 ) ;
#14913=ORIENTED_EDGE ( 'NONE', *, *, #9591, .F. ) ;
#14917=EDGE_LOOP ( 'NONE', ( #7775, #7845, #12285, #12242 ) ) ;
#14927=CARTESIAN_POINT ( 'NONE',  ( -25.00000000000000000, 53.00000000000000711, 30.00000000000000000 ) ) ;
#14939=CARTESIAN_POINT ( 'NONE',  ( -25.00000000000000000, 53.00000000000000711, -50.00000000000000000 ) ) ;
#14940=CARTESIAN_POINT ( 'NONE',  ( -40.00000000000000711, 110.0000000000000000, 19.99999999999999645 ) ) ;
#14943=CARTESIAN_POINT ( 'NONE',  ( -25.00000000000000711, 110.0000000000000000, -6.000000000000001776 ) ) ;
#14944=FACE_OUTER_BOUND ( 'NONE', #15102, .T. ) ;
#14961=DIRECTION ( 'NONE',  ( 0.000000000000000000, -1.000000000000000000, 0.000000000000000000 ) ) ;
#14962=CARTESIAN_POINT ( 'NONE',  ( -41.00000000000000711, 110.0000000000000000, -11.50000000000000355 ) ) ;
#14963=CARTESIAN_POINT ( 'NONE',  ( -24.00000000000000000, 53.00000000000000711, 8.000000000000000000 ) ) ;
#14966=EDGE_CURVE ( 'NONE', #14005, #6936, #7812, .T. ) ;
#14968=ORIENTED_EDGE ( 'NONE', *, *, #1295, .T. ) ;
#14971=CARTESIAN_POINT ( 'NONE',  ( -41.00000000000000711, 110.0000000000000000, -24.49999999999999645 ) ) ;
#14979=EDGE_LOOP ( 'NONE', ( #11177, #11620, #3231, #1651 ) ) ;
#14988=EDGE_CURVE ( 'NONE', #1673, #7148, #12409, .T. ) ;
#14989=LINE ( 'NONE', #14600, #15517 ) ;
#14992=ORIENTED_EDGE ( 'NONE', *, *, #18936, .T. ) ;
#15002=CARTESIAN_POINT ( 'NONE',  ( -32.50000000000000000, 53.00000000000000711, -35.00000000000000000 ) ) ;
#15005=VECTOR ( 'NONE', #18328, 1000.000000000000000 ) ;
#15006=CARTESIAN_POINT ( 'NONE',  ( -41.00000000000000711, 53.00000000000000711, 20.00000000000000000 ) ) ;
#15010=CARTESIAN_POINT ( 'NONE',  ( -41.00000000000000711, 53.00000000000000711, -12.50000000000000000 ) ) ;
#15013=PLANE ( 'NONE',  #1931 ) ;
#15014=VECTOR ( 'NONE', #592, 1000.000000000000000 ) ;
#15016=LINE ( 'NONE', #7366, #3509 ) ;
#15019=( NAMED_UNIT ( * ) SI_UNIT ( $, .STERADIAN. ) SOLID_ANGLE_UNIT ( ) );
#15024=LINE ( 'NONE', #14927, #9579 ) ;
#15030=VERTEX_POINT ( 'NONE', #9468 ) ;
#15032=DIRECTION ( 'NONE',  ( 0.000000000000000000, -1.000000000000000000, 0.000000000000000000 ) ) ;
#15038=VECTOR ( 'NONE', #18892, 1000.000000000000000 ) ;
#15041=ADVANCED_FACE ( 'NONE', ( #10636 ), #18211, .F. ) ;
#15044=VECTOR ( 'NONE', #19345, 1000.000000000000000 ) ;
#15045=ORIENTED_EDGE ( 'NONE', *, *, #12010, .T. ) ;
#15053=VECTOR ( 'NONE', #3449, 1000.000000000000000 ) ;
#15054=DIRECTION ( 'NONE',  ( 0.000000000000000000, 0.000000000000000000, -1.000000000000000000 ) ) ;
#15060=EDGE_CURVE ( 'NONE', #10380, #12337, #15259, .T. ) ;
#15067=CARTESIAN_POINT ( 'NONE',  ( -25.00000000000000711, 53.00000000000000711, -30.99999999999999645 ) ) ;
#15071=EDGE_CURVE ( 'NONE', #1832, #17252, #3096, .T. ) ;
#15079=DIRECTION ( 'NONE',  ( 0.000000000000000000, 0.000000000000000000, -1.000000000000000000 ) ) ;
#15088=LINE ( 'NONE', #10459, #3837 ) ;
#15089=ORIENTED_EDGE ( 'NONE', *, *, #1135, .F. ) ;
#15091=CARTESIAN_POINT ( 'NONE',  ( -41.00000000000000711, 110.0000000000000000, -11.50000000000000000 ) ) ;
#15094=LINE ( 'NONE', #10466, #12546 ) ;
#15102=EDGE_LOOP ( 'NONE', ( #4443, #6778, #4351, #12255 ) ) ;
#15103=ORIENTED_EDGE ( 'NONE', *, *, #9023, .T. ) ;
#15114=CARTESIAN_POINT ( 'NONE',  ( -41.00000000000000711, 110.0000000000000000, 27.50000000000000000 ) ) ;
#15117=LINE ( 'NONE', #10396, #11011 ) ;
#15123=EDGE_CURVE ( 'NONE', #13902, #17838, #5258, .T. ) ;
#15125=ORIENTED_EDGE ( 'NONE', *, *, #3494, .F. ) ;
#15128=LINE ( 'NONE', #2340, #3814 ) ;
#15139=CARTESIAN_POINT ( 'NONE',  ( -40.00000000000000000, 53.00000000000000711, 30.00000000000000000 ) ) ;
#15140=EDGE_CURVE ( 'NONE', #76, #11826, #8106, .T. ) ;
#15149=EDGE_CURVE ( 'NONE', #18134, #3857, #12882, .T. ) ;
#15152=EDGE_CURVE ( 'NONE', #11826, #1662, #1029, .T. ) ;
#15157=EDGE_CURVE ( 'NONE', #17823, #7137, #14076, .T. ) ;
#15161=DIRECTION ( 'NONE',  ( 0.000000000000000000, 0.000000000000000000, -1.000000000000000000 ) ) ;
#15163=DIRECTION ( 'NONE',  ( 1.000000000000000000, -0.000000000000000000, -0.000000000000000000 ) ) ;
#15165=AXIS2_PLACEMENT_3D ( 'NONE', #15139, #6029, #13462 ) ;
#15172=ORIENTED_EDGE ( 'NONE', *, *, #9886, .F. ) ;
#15173=ORIENTED_EDGE ( 'NONE', *, *, #11069, .T. ) ;
#15190=CARTESIAN_POINT ( 'NONE',  ( -41.00000000000000711, 53.00000000000000711, 1.500000000000001332 ) ) ;
#15210=EDGE_LOOP ( 'NONE', ( #16666, #11237, #4836, #17828 ) ) ;
#15213=FACE_OUTER_BOUND ( 'NONE', #5981, .T. ) ;
#15216=VECTOR ( 'NONE', #15079, 1000.000000000000000 ) ;
#15218=LINE ( 'NONE', #6299, #14413 ) ;
#15220=DIRECTION ( 'NONE',  ( -1.000000000000000000, 0.000000000000000000, -0.000000000000000000 ) ) ;
#15231=PLANE ( 'NONE',  #5313 ) ;
#15235=CARTESIAN_POINT ( 'NONE',  ( -41.00000000000000711, 53.00000000000000711, -12.50000000000000000 ) ) ;
#15237=VECTOR ( 'NONE', #18692, 1000.000000000000000 ) ;
#15240=VERTEX_POINT ( 'NONE', #15834 ) ;
#15246=COLOUR_RGB ( '', 0.72549020, 0.75294118, 0.79215686) ;
#15247=AXIS2_PLACEMENT_3D ( 'NONE', #2587, #11398, #8476 ) ;
#15257=LINE ( 'NONE', #10928, #18697 ) ;
#15259=LINE ( 'NONE', #10837, #7692 ) ;
#15262=ORIENTED_EDGE ( 'NONE', *, *, #16694, .T. ) ;
#15269=CARTESIAN_POINT ( 'NONE',  ( -41.00000000000000711, 53.00000000000000711, -19.00000000000000000 ) ) ;
#15277=ORIENTED_EDGE ( 'NONE', *, *, #14337, .F. ) ;
#15279=DIRECTION ( 'NONE',  ( 0.000000000000000000, 0.000000000000000000, -1.000000000000000000 ) ) ;
#15280=DIRECTION ( 'NONE',  ( -0.000000000000000000, -0.000000000000000000, -1.000000000000000000 ) ) ;
#15282=EDGE_CURVE ( 'NONE', #12144, #14297, #12781, .T. ) ;
#15286=VERTEX_POINT ( 'NONE', #5927 ) ;
#15291=ORIENTED_EDGE ( 'NONE', *, *, #7786, .T. ) ;
#15299=ORIENTED_EDGE ( 'NONE', *, *, #1878, .F. ) ;
#15301=ORIENTED_EDGE ( 'NONE', *, *, #17, .F. ) ;
#15303=DIRECTION ( 'NONE',  ( 0.000000000000000000, -1.000000000000000000, -0.000000000000000000 ) ) ;
#15305=DIRECTION ( 'NONE',  ( -1.000000000000000000, 0.000000000000000000, -0.000000000000000000 ) ) ;
#15306=EDGE_CURVE ( 'NONE', #14701, #1350, #14549, .T. ) ;
#15307=LINE ( 'NONE', #13731, #530 ) ;
#15311=FACE_OUTER_BOUND ( 'NONE', #10617, .T. ) ;
#15323=ORIENTED_EDGE ( 'NONE', *, *, #12010, .F. ) ;
#15330=LINE ( 'NONE', #2000, #2023 ) ;
#15333=VECTOR ( 'NONE', #15032, 1000.000000000000000 ) ;
#15334=VECTOR ( 'NONE', #8902, 1000.000000000000000 ) ;
#15338=AXIS2_PLACEMENT_3D ( 'NONE', #864, #12725, #6843 ) ;
#15344=LINE ( 'NONE', #15445, #14863 ) ;
#15346=AXIS2_PLACEMENT_3D ( 'NONE', #15967, #6947, #9787 ) ;
#15353=DIRECTION ( 'NONE',  ( -0.000000000000000000, -0.000000000000000000, -1.000000000000000000 ) ) ;
#15358=VECTOR ( 'NONE', #19328, 1000.000000000000000 ) ;
#15359=EDGE_LOOP ( 'NONE', ( #4243, #480, #17453, #767 ) ) ;
#15370=VECTOR ( 'NONE', #16357, 1000.000000000000000 ) ;
#15375=LINE ( 'NONE', #4699, #11890 ) ;
#15378=ADVANCED_FACE ( 'NONE', ( #17789 ), #1214, .T. ) ;
#15379=LINE ( 'NONE', #18425, #15005 ) ;
#15381=EDGE_CURVE ( 'NONE', #2609, #12636, #17593, .T. ) ;
#15387=ORIENTED_EDGE ( 'NONE', *, *, #18853, .T. ) ;
#15390=ORIENTED_EDGE ( 'NONE', *, *, #2810, .F. ) ;
#15393=ORIENTED_EDGE ( 'NONE', *, *, #10084, .T. ) ;
#15403=EDGE_CURVE ( 'NONE', #13814, #11652, #11497, .T. ) ;
#15406=ORIENTED_EDGE ( 'NONE', *, *, #12471, .T. ) ;
#15410=CARTESIAN_POINT ( 'NONE',  ( -41.00000000000000711, 110.0000000000000000, 6.999999999999999112 ) ) ;
#15411=DIRECTION ( 'NONE',  ( 0.000000000000000000, 0.000000000000000000, 1.000000000000000000 ) ) ;
#15413=VECTOR ( 'NONE', #10735, 1000.000000000000000 ) ;
#15414=EDGE_CURVE ( 'NONE', #13282, #6823, #11694, .T. ) ;
#15415=CARTESIAN_POINT ( 'NONE',  ( -41.00000000000000711, 53.00000000000000711, -11.50000000000000000 ) ) ;
#15423=PLANE ( 'NONE',  #1465 ) ;
#15431=ORIENTED_EDGE ( 'NONE', *, *, #64, .F. ) ;
#15434=LINE ( 'NONE', #1906, #17563 ) ;
#15437=LINE ( 'NONE', #9339, #10031 ) ;
#15438=PLANE ( 'NONE',  #7391 ) ;
#15439=ORIENTED_EDGE ( 'NONE', *, *, #14558, .F. ) ;
#15443=CARTESIAN_POINT ( 'NONE',  ( -41.00000000000000000, 52.00000000000000711, -50.00000000000000000 ) ) ;
#15445=CARTESIAN_POINT ( 'NONE',  ( -41.00000000000000711, 53.00000000000000711, -30.99999999999999645 ) ) ;
#15454=LINE ( 'NONE', #9178, #16131 ) ;
#15468=EDGE_CURVE ( 'NONE', #16704, #291, #8759, .T. ) ;
#15479=ORIENTED_EDGE ( 'NONE', *, *, #14542, .T. ) ;
#15488=VECTOR ( 'NONE', #16205, 1000.000000000000000 ) ;
#15490=DIRECTION ( 'NONE',  ( 0.000000000000000000, 0.000000000000000000, -1.000000000000000000 ) ) ;
#15500=CARTESIAN_POINT ( 'NONE',  ( -24.00000000000000711, 53.00000000000000711, 13.50000000000000000 ) ) ;
#15501=CARTESIAN_POINT ( 'NONE',  ( -24.00000000000000000, 53.00000000000000711, 30.00000000000000000 ) ) ;
#15503=PLANE ( 'NONE',  #12215 ) ;
#15511=EDGE_CURVE ( 'NONE', #5957, #2980, #13065, .T. ) ;
#15512=ORIENTED_EDGE ( 'NONE', *, *, #13926, .F. ) ;
#15517=VECTOR ( 'NONE', #1167, 1000.000000000000000 ) ;
#15518=CARTESIAN_POINT ( 'NONE',  ( -40.00000000000000000, 53.00000000000000711, -12.50000000000000000 ) ) ;
#15519=VERTEX_POINT ( 'NONE', #9448 ) ;
#15524=DIRECTION ( 'NONE',  ( 0.000000000000000000, 1.000000000000000000, 0.000000000000000000 ) ) ;
#15526=LINE ( 'NONE', #6611, #3799 ) ;
#15530=ADVANCED_FACE ( 'NONE', ( #18387 ), #46, .F. ) ;
#15533=DIRECTION ( 'NONE',  ( -1.156482317317871478E-16, 1.000000000000000000, 0.000000000000000000 ) ) ;
#15534=VECTOR ( 'NONE', #10848, 1000.000000000000000 ) ;
#15560=DIRECTION ( 'NONE',  ( 0.000000000000000000, -1.000000000000000000, -0.000000000000000000 ) ) ;
#15572=ADVANCED_FACE ( 'NONE', ( #1520 ), #16514, .T. ) ;
#15591=VERTEX_POINT ( 'NONE', #9056 ) ;
#15594=LINE ( 'NONE', #11733, #2797 ) ;
#15598=CARTESIAN_POINT ( 'NONE',  ( -24.00000000000000000, 53.00000000000000711, -37.50000000000000711 ) ) ;
#15600=VERTEX_POINT ( 'NONE', #13657 ) ;
#15614=VECTOR ( 'NONE', #1929, 1000.000000000000000 ) ;
#15617=EDGE_CURVE ( 'NONE', #12352, #15030, #7488, .T. ) ;
#15618=CARTESIAN_POINT ( 'NONE',  ( -32.50000000000000000, 53.00000000000000711, 17.64999999999999147 ) ) ;
#15620=FACE_OUTER_BOUND ( 'NONE', #9197, .T. ) ;
#15621=VECTOR ( 'NONE', #1844, 1000.000000000000000 ) ;
#15629=CARTESIAN_POINT ( 'NONE',  ( -41.00000000000000711, 53.00000000000000711, -25.50000000000000000 ) ) ;
#15632=VECTOR ( 'NONE', #4306, 1000.000000000000000 ) ;
#15638=LINE ( 'NONE', #738, #11509 ) ;
#15643=EDGE_CURVE ( 'NONE', #7955, #12973, #16906, .T. ) ;
#15646=VERTEX_POINT ( 'NONE', #17984 ) ;
#15656=ORIENTED_EDGE ( 'NONE', *, *, #1479, .T. ) ;
#15666=CARTESIAN_POINT ( 'NONE',  ( -41.00000000000000711, 110.0000000000000000, -5.000000000000000888 ) ) ;
#15670=ORIENTED_EDGE ( 'NONE', *, *, #14652, .F. ) ;
#15675=ORIENTED_EDGE ( 'NONE', *, *, #15747, .F. ) ;
#15679=VECTOR ( 'NONE', #8885, 1000.000000000000000 ) ;
#15682=DIRECTION ( 'NONE',  ( 0.000000000000000000, -1.000000000000000000, -0.000000000000000000 ) ) ;
#15687=ORIENTED_EDGE ( 'NONE', *, *, #5808, .F. ) ;
#15692=CARTESIAN_POINT ( 'NONE',  ( -40.00000000000000711, 110.0000000000000000, -25.49999999999999645 ) ) ;
#15701=ORIENTED_EDGE ( 'NONE', *, *, #18148, .F. ) ;
#15705=ORIENTED_EDGE ( 'NONE', *, *, #6024, .T. ) ;
#15711=EDGE_LOOP ( 'NONE', ( #12439, #7516, #17722, #3617 ) ) ;
#15722=FACE_BOUND ( 'NONE', #18139, .T. ) ;
#15724=FACE_OUTER_BOUND ( 'NONE', #3106, .T. ) ;
#15729=VECTOR ( 'NONE', #17108, 1000.000000000000000 ) ;
#15747=EDGE_CURVE ( 'NONE', #11338, #1767, #17194, .T. ) ;
#15749=ADVANCED_FACE ( 'NONE', ( #15620 ), #14152, .T. ) ;
#15751=CARTESIAN_POINT ( 'NONE',  ( -41.00000000000000000, 52.00000000000000711, 30.00000000000000000 ) ) ;
#15755=ORIENTED_EDGE ( 'NONE', *, *, #12857, .T. ) ;
#15761=CARTESIAN_POINT ( 'NONE',  ( -24.00000000000000000, 53.00000000000000711, 30.00000000000000000 ) ) ;
#15765=ORIENTED_EDGE ( 'NONE', *, *, #11409, .T. ) ;
#15766=ORIENTED_EDGE ( 'NONE', *, *, #18100, .F. ) ;
#15767=ADVANCED_FACE ( 'NONE', ( #8088 ), #15438, .T. ) ;
#15770=ORIENTED_EDGE ( 'NONE', *, *, #11308, .T. ) ;
#15776=FACE_OUTER_BOUND ( 'NONE', #2619, .T. ) ;
#15782=DIRECTION ( 'NONE',  ( -1.156482317317871478E-16, 1.000000000000000000, 0.000000000000000000 ) ) ;
#15789=LINE ( 'NONE', #15977, #13959 ) ;
#15796=ORIENTED_EDGE ( 'NONE', *, *, #8394, .F. ) ;
#15803=PLANE ( 'NONE',  #4691 ) ;
#15814=ORIENTED_EDGE ( 'NONE', *, *, #6424, .F. ) ;
#15822=DIRECTION ( 'NONE',  ( -1.000000000000000000, 0.000000000000000000, -0.000000000000000000 ) ) ;
#15830=VECTOR ( 'NONE', #9090, 1000.000000000000000 ) ;
#15834=CARTESIAN_POINT ( 'NONE',  ( -25.00000000000000000, 110.0000000000000000, -5.000000000000004441 ) ) ;
#15847=DIRECTION ( 'NONE',  ( 1.000000000000000000, -0.000000000000000000, -0.000000000000000000 ) ) ;
#15861=ORIENTED_EDGE ( 'NONE', *, *, #6743, .T. ) ;
#15862=ORIENTED_EDGE ( 'NONE', *, *, #17741, .T. ) ;
#15874=ORIENTED_EDGE ( 'NONE', *, *, #8436, .F. ) ;
#15875=CARTESIAN_POINT ( 'NONE',  ( -40.00000000000000711, 113.0000000000000000, 8.000000000000000000 ) ) ;
#15881=LINE ( 'NONE', #2442, #17394 ) ;
#15884=ORIENTED_EDGE ( 'NONE', *, *, #15414, .T. ) ;
#15890=ORIENTED_EDGE ( 'NONE', *, *, #3136, .T. ) ;
#15895=VERTEX_POINT ( 'NONE', #17463 ) ;
#15899=LINE ( 'NONE', #2463, #12561 ) ;
#15907=UNCERTAINTY_MEASURE_WITH_UNIT (LENGTH_MEASURE( 1.000000000000000082E-05 ), #14288, 'distance_accuracy_value', 'NONE');
#15908=SHAPE_REPRESENTATION ( 'Heating Element & carriage', ( #1791 ), #2707 ) ;
#15915=EDGE_CURVE ( 'NONE', #16834, #10481, #8731, .T. ) ;
#15919=CARTESIAN_POINT ( 'NONE',  ( -32.50000000000000000, 53.00000000000000711, -32.35000000000001563 ) ) ;
#15920=DIRECTION ( 'NONE',  ( -0.000000000000000000, -0.000000000000000000, -1.000000000000000000 ) ) ;
#15944=CARTESIAN_POINT ( 'NONE',  ( -41.00000000000000711, 110.0000000000000000, -37.50000000000000711 ) ) ;
#15947=PLANE ( 'NONE',  #4261 ) ;
#15952=VECTOR ( 'NONE', #7681, 1000.000000000000000 ) ;
#15956=ORIENTED_EDGE ( 'NONE', *, *, #11695, .T. ) ;
#15962=CARTESIAN_POINT ( 'NONE',  ( -24.00000000000000000, 53.00000000000000711, 30.00000000000000000 ) ) ;
#15966=ORIENTED_EDGE ( 'NONE', *, *, #8174, .F. ) ;
#15967=CARTESIAN_POINT ( 'NONE',  ( -41.00000000000000711, 110.0000000000000000, -44.00000000000000000 ) ) ;
#15975=EDGE_CURVE ( 'NONE', #10054, #1553, #1392, .T. ) ;
#15976=DIRECTION ( 'NONE',  ( 0.000000000000000000, -1.000000000000000000, 0.000000000000000000 ) ) ;
#15977=CARTESIAN_POINT ( 'NONE',  ( -41.00000000000000711, 113.0000000000000000, -50.00000000000000000 ) ) ;
#15980=ORIENTED_EDGE ( 'NONE', *, *, #2062, .F. ) ;
#15981=ORIENTED_EDGE ( 'NONE', *, *, #6865, .F. ) ;
#15982=EDGE_LOOP ( 'NONE', ( #3763, #15966, #18310, #8790 ) ) ;
#15984=LINE ( 'NONE', #3835, #9907 ) ;
#15985=VECTOR ( 'NONE', #13285, 1000.000000000000000 ) ;
#15986=ORIENTED_EDGE ( 'NONE', *, *, #12356, .F. ) ;
#15988=VECTOR ( 'NONE', #3357, 1000.000000000000000 ) ;
#15991=DIRECTION ( 'NONE',  ( 0.000000000000000000, 0.000000000000000000, -1.000000000000000000 ) ) ;
#16006=FACE_BOUND ( 'NONE', #17917, .T. ) ;
#16009=DIRECTION ( 'NONE',  ( 0.000000000000000000, 0.000000000000000000, -1.000000000000000000 ) ) ;
#16026=DIRECTION ( 'NONE',  ( 0.000000000000000000, 1.000000000000000000, 0.000000000000000000 ) ) ;
#16027=CYLINDRICAL_SURFACE ( 'NONE', #15247, 2.649999999999992806 ) ;
#16029=CARTESIAN_POINT ( 'NONE',  ( -41.00000000000000711, 110.0000000000000000, -30.99999999999999645 ) ) ;
#16031=ADVANCED_FACE ( 'NONE', ( #9424 ), #12562, .T. ) ;
#16043=DIRECTION ( 'NONE',  ( -0.000000000000000000, 1.000000000000000000, -0.000000000000000000 ) ) ;
#16047=ORIENTED_EDGE ( 'NONE', *, *, #12486, .T. ) ;
#16058=CARTESIAN_POINT ( 'NONE',  ( -41.00000000000000711, 53.00000000000000711, 20.00000000000000000 ) ) ;
#16060=CARTESIAN_POINT ( 'NONE',  ( -25.00000000000000000, 53.00000000000000711, 30.00000000000000000 ) ) ;
#16063=CARTESIAN_POINT ( 'NONE',  ( -40.00000000000000711, 53.00000000000000711, -18.00000000000000000 ) ) ;
#16074=LINE ( 'NONE', #12836, #824 ) ;
#16078=LINE ( 'NONE', #14138, #3103 ) ;
#16083=DIRECTION ( 'NONE',  ( 0.000000000000000000, 0.000000000000000000, 1.000000000000000000 ) ) ;
#16085=CARTESIAN_POINT ( 'NONE',  ( -40.00000000000000711, 113.0000000000000000, 13.49999999999999822 ) ) ;
#16086=CARTESIAN_POINT ( 'NONE',  ( -41.00000000000000711, 53.00000000000000711, -12.50000000000000000 ) ) ;
#16091=EDGE_CURVE ( 'NONE', #8804, #17825, #9612, .T. ) ;
#16110=CYLINDRICAL_SURFACE ( 'NONE', #7512, 2.649999999999992806 ) ;
#16111=LINE ( 'NONE', #39, #599 ) ;
#16113=ADVANCED_FACE ( 'NONE', ( #9704 ), #12363, .F. ) ;
#16117=LINE ( 'NONE', #9835, #7986 ) ;
#16121=ORIENTED_EDGE ( 'NONE', *, *, #14904, .T. ) ;
#16131=VECTOR ( 'NONE', #15163, 1000.000000000000000 ) ;
#16138=DIRECTION ( 'NONE',  ( 0.000000000000000000, 0.000000000000000000, -1.000000000000000000 ) ) ;
#16144=ORIENTED_EDGE ( 'NONE', *, *, #18974, .T. ) ;
#16154=ORIENTED_EDGE ( 'NONE', *, *, #2439, .T. ) ;
#16155=DIRECTION ( 'NONE',  ( 0.000000000000000000, 0.000000000000000000, 1.000000000000000000 ) ) ;
#16161=CIRCLE ( 'NONE', #12413, 2.649999999999985700 ) ;
#16167=EDGE_LOOP ( 'NONE', ( #7023, #4300, #2649, #8241, #11095, #8761, #16144, #15675, #12445, #13589, #2638, #15512, #494, #11941, #10666, #18076, #5723, #4006, #3367, #3465, #3820, #18365, #17488, #950, #5503, #7221, #7152, #17330, #2142, #10790, #15173, #8993, #3810, #15045, #17629, #12042, #1735, #3436, #16753, #2444, #13863, #16370, #9011, #9180, #15125, #14291, #8827, #5146, #5540, #1893, #18909, #14578 ) ) ;
#16180=ORIENTED_EDGE ( 'NONE', *, *, #13911, .T. ) ;
#16182=EDGE_LOOP ( 'NONE', ( #17614, #8683, #15986, #6158 ) ) ;
#16194=ORIENTED_EDGE ( 'NONE', *, *, #11793, .T. ) ;
#16202=LINE ( 'NONE', #14735, #15952 ) ;
#16204=ADVANCED_FACE ( 'NONE', ( #13633 ), #9224, .T. ) ;
#16205=DIRECTION ( 'NONE',  ( 0.000000000000000000, 1.000000000000000000, 0.000000000000000000 ) ) ;
#16219=EDGE_CURVE ( 'NONE', #10251, #9405, #3151, .T. ) ;
#16220=ADVANCED_FACE ( 'NONE', ( #18359 ), #3252, .T. ) ;
#16225=EDGE_CURVE ( 'NONE', #6936, #6193, #15307, .T. ) ;
#16233=ORIENTED_EDGE ( 'NONE', *, *, #14542, .F. ) ;
#16244=DIRECTION ( 'NONE',  ( 0.000000000000000000, -0.000000000000000000, 1.000000000000000000 ) ) ;
#16261=EDGE_LOOP ( 'NONE', ( #2244, #2531 ) ) ;
#16262=VERTEX_POINT ( 'NONE', #218 ) ;
#16268=ORIENTED_EDGE ( 'NONE', *, *, #5203, .T. ) ;
#16273=ORIENTED_EDGE ( 'NONE', *, *, #8794, .F. ) ;
#16277=ORIENTED_EDGE ( 'NONE', *, *, #3988, .T. ) ;
#16283=VECTOR ( 'NONE', #11092, 1000.000000000000000 ) ;
#16284=DIRECTION ( 'NONE',  ( 1.000000000000000000, -0.000000000000000000, -0.000000000000000000 ) ) ;
#16288=VECTOR ( 'NONE', #6397, 1000.000000000000000 ) ;
#16319=VECTOR ( 'NONE', #7985, 1000.000000000000000 ) ;
#16333=LINE ( 'NONE', #13482, #13108 ) ;
#16335=AXIS2_PLACEMENT_3D ( 'NONE', #11902, #1425, #10423 ) ;
#16346=CARTESIAN_POINT ( 'NONE',  ( -24.00000000000000711, 53.00000000000000711, 8.000000000000000000 ) ) ;
#16355=ORIENTED_EDGE ( 'NONE', *, *, #12708, .T. ) ;
#16357=DIRECTION ( 'NONE',  ( 1.000000000000000000, -0.000000000000000000, -0.000000000000000000 ) ) ;
#16367=CARTESIAN_POINT ( 'NONE',  ( -32.50000000000000000, 53.00000000000000711, -37.64999999999999147 ) ) ;
#16369=VERTEX_POINT ( 'NONE', #7411 ) ;
#16370=ORIENTED_EDGE ( 'NONE', *, *, #8898, .T. ) ;
#16374=ORIENTED_EDGE ( 'NONE', *, *, #3571, .T. ) ;
#16383=CARTESIAN_POINT ( 'NONE',  ( -41.00000000000000711, 53.00000000000000711, -11.50000000000000000 ) ) ;
#16384=VERTEX_POINT ( 'NONE', #14962 ) ;
#16385=FACE_OUTER_BOUND ( 'NONE', #16749, .T. ) ;
#16392=CARTESIAN_POINT ( 'NONE',  ( -25.00000000000000000, 53.00000000000000711, 30.00000000000000000 ) ) ;
#16399=FACE_OUTER_BOUND ( 'NONE', #13697, .T. ) ;
#16400=ORIENTED_EDGE ( 'NONE', *, *, #1400, .F. ) ;
#16408=CARTESIAN_POINT ( 'NONE',  ( -24.00000000000000711, 110.0000000000000000, -30.99999999999999645 ) ) ;
#16411=FACE_OUTER_BOUND ( 'NONE', #1241, .T. ) ;
#16422=ADVANCED_FACE ( 'NONE', ( #16637 ), #6242, .T. ) ;
#16425=PLANE ( 'NONE',  #3410 ) ;
#16434=CARTESIAN_POINT ( 'NONE',  ( -41.00000000000000711, 110.0000000000000000, 8.000000000000000000 ) ) ;
#16439=LINE ( 'NONE', #13387, #15985 ) ;
#16440=EDGE_LOOP ( 'NONE', ( #1740, #10839, #2863, #9410 ) ) ;
#16443=LINE ( 'NONE', #18019, #11738 ) ;
#16452=CARTESIAN_POINT ( 'NONE',  ( -25.00000000000000711, 110.0000000000000000, -12.50000000000000000 ) ) ;
#16453=EDGE_CURVE ( 'NONE', #3017, #6733, #13278, .T. ) ;
#16456=LINE ( 'NONE', #4703, #12500 ) ;
#16457=ADVANCED_FACE ( 'NONE', ( #19375 ), #7808, .T. ) ;
#16460=CARTESIAN_POINT ( 'NONE',  ( -25.00000000000000711, 53.00000000000000711, -19.00000000000000000 ) ) ;
#16461=VECTOR ( 'NONE', #3055, 1000.000000000000000 ) ;
#16469=ORIENTED_EDGE ( 'NONE', *, *, #15381, .T. ) ;
#16480=EDGE_CURVE ( 'NONE', #15286, #1273, #11123, .T. ) ;
#16485=LINE ( 'NONE', #16085, #17245 ) ;
#16487=CARTESIAN_POINT ( 'NONE',  ( -24.00000000000000000, 53.00000000000000711, -5.000000000000004441 ) ) ;
#16503=ORIENTED_EDGE ( 'NONE', *, *, #17741, .F. ) ;
#16510=EDGE_CURVE ( 'NONE', #11826, #8366, #17119, .T. ) ;
#16514=PLANE ( 'NONE',  #6143 ) ;
#16527=DIRECTION ( 'NONE',  ( -1.156482317317871478E-16, 1.000000000000000000, 0.000000000000000000 ) ) ;
#16528=CARTESIAN_POINT ( 'NONE',  ( -25.00000000000000000, 53.00000000000000711, -31.00000000000000000 ) ) ;
#16531=DIRECTION ( 'NONE',  ( 0.000000000000000000, 0.000000000000000000, 1.000000000000000000 ) ) ;
#16532=CARTESIAN_POINT ( 'NONE',  ( -41.00000000000000711, 53.00000000000000711, -24.49999999999999645 ) ) ;
#16539=VERTEX_POINT ( 'NONE', #11026 ) ;
#16547=EDGE_CURVE ( 'NONE', #184, #10051, #12690, .T. ) ;
#16551=DIRECTION ( 'NONE',  ( -1.156482317317871478E-16, 1.000000000000000000, 0.000000000000000000 ) ) ;
#16552=ORIENTED_EDGE ( 'NONE', *, *, #14337, .T. ) ;
#16555=EDGE_CURVE ( 'NONE', #6193, #1050, #15257, .T. ) ;
#16557=CARTESIAN_POINT ( 'NONE',  ( -41.00000000000000711, 110.0000000000000000, -18.00000000000000355 ) ) ;
#16558=EDGE_CURVE ( 'NONE', #12791, #11, #3391, .T. ) ;
#16572=LINE ( 'NONE', #3240, #16913 ) ;
#16573=ORIENTED_EDGE ( 'NONE', *, *, #10597, .T. ) ;
#16580=EDGE_CURVE ( 'NONE', #1832, #11, #3492, .T. ) ;
#16583=VECTOR ( 'NONE', #8265, 1000.000000000000000 ) ;
#16586=DIRECTION ( 'NONE',  ( 0.000000000000000000, 0.000000000000000000, -1.000000000000000000 ) ) ;
#16601=DIRECTION ( 'NONE',  ( 0.000000000000000000, 0.000000000000000000, 1.000000000000000000 ) ) ;
#16602=ORIENTED_EDGE ( 'NONE', *, *, #5806, .F. ) ;
#16603=VECTOR ( 'NONE', #4199, 1000.000000000000000 ) ;
#16612=ADVANCED_FACE ( 'NONE', ( #18968 ), #16027, .F. ) ;
#16613=LINE ( 'NONE', #3179, #12945 ) ;
#16614=CARTESIAN_POINT ( 'NONE',  ( -41.00000000000000711, 110.0000000000000000, 14.50000000000000000 ) ) ;
#16619=VECTOR ( 'NONE', #18059, 1000.000000000000000 ) ;
#16624=AXIS2_PLACEMENT_3D ( 'NONE', #1368, #7337, #14892 ) ;
#16631=AXIS2_PLACEMENT_3D ( 'NONE', #6846, #12729, #18725 ) ;
#16634=CARTESIAN_POINT ( 'NONE',  ( -41.00000000000000711, 110.0000000000000000, -25.50000000000000000 ) ) ;
#16637=FACE_OUTER_BOUND ( 'NONE', #11649, .T. ) ;
#16642=VERTEX_POINT ( 'NONE', #19162 ) ;
#16643=ORIENTED_EDGE ( 'NONE', *, *, #18834, .T. ) ;
#16656=ORIENTED_EDGE ( 'NONE', *, *, #7318, .T. ) ;
#16658=ORIENTED_EDGE ( 'NONE', *, *, #7786, .F. ) ;
#16665=ORIENTED_EDGE ( 'NONE', *, *, #5921, .F. ) ;
#16666=ORIENTED_EDGE ( 'NONE', *, *, #11425, .T. ) ;
#16670=AXIS2_PLACEMENT_3D ( 'NONE', #9934, #11502, #19068 ) ;
#16677=DIRECTION ( 'NONE',  ( 0.000000000000000000, 0.000000000000000000, 1.000000000000000000 ) ) ;
#16683=VERTEX_POINT ( 'NONE', #3968 ) ;
#16694=EDGE_CURVE ( 'NONE', #184, #9810, #12880, .T. ) ;
#16704=VERTEX_POINT ( 'NONE', #6813 ) ;
#16714=UNCERTAINTY_MEASURE_WITH_UNIT (LENGTH_MEASURE( 1.000000000000000082E-05 ), #12339, 'distance_accuracy_value', 'NONE');
#16721=EDGE_CURVE ( 'NONE', #11533, #853, #16117, .T. ) ;
#16726=DIRECTION ( 'NONE',  ( 0.000000000000000000, -1.000000000000000000, 0.000000000000000000 ) ) ;
#16737=ORIENTED_EDGE ( 'NONE', *, *, #12173, .T. ) ;
#16749=EDGE_LOOP ( 'NONE', ( #14185, #15393, #14132, #1421 ) ) ;
#16753=ORIENTED_EDGE ( 'NONE', *, *, #10824, .T. ) ;
#16758=DIRECTION ( 'NONE',  ( 1.000000000000000000, -0.000000000000000000, -0.000000000000000000 ) ) ;
#16766=VECTOR ( 'NONE', #15411, 1000.000000000000000 ) ;
#16773=ORIENTED_EDGE ( 'NONE', *, *, #2886, .F. ) ;
#16781=DIRECTION ( 'NONE',  ( 0.000000000000000000, 0.000000000000000000, 1.000000000000000000 ) ) ;
#16785=DIRECTION ( 'NONE',  ( -1.000000000000000000, 0.000000000000000000, -0.000000000000000000 ) ) ;
#16792=VERTEX_POINT ( 'NONE', #7486 ) ;
#16795=VECTOR ( 'NONE', #11030, 1000.000000000000000 ) ;
#16799=CARTESIAN_POINT ( 'NONE',  ( -24.00000000000000000, 110.0000000000000000, 13.50000000000000178 ) ) ;
#16803=ADVANCED_FACE ( 'NONE', ( #11692, #2881, #16411 ), #11989, .T. ) ;
#16811=DIRECTION ( 'NONE',  ( 0.000000000000000000, 0.000000000000000000, -1.000000000000000000 ) ) ;
#16812=ORIENTED_EDGE ( 'NONE', *, *, #4129, .T. ) ;
#16815=EDGE_CURVE ( 'NONE', #4659, #7863, #5831, .T. ) ;
#16820=DIRECTION ( 'NONE',  ( -1.000000000000000000, 0.000000000000000000, -0.000000000000000000 ) ) ;
#16829=DIRECTION ( 'NONE',  ( 0.000000000000000000, 1.000000000000000000, 0.000000000000000000 ) ) ;
#16830=DIRECTION ( 'NONE',  ( 0.000000000000000000, 1.000000000000000000, 0.000000000000000000 ) ) ;
#16834=VERTEX_POINT ( 'NONE', #10415 ) ;
#16837=EDGE_CURVE ( 'NONE', #10481, #7135, #16613, .T. ) ;
#16840=ORIENTED_EDGE ( 'NONE', *, *, #7360, .F. ) ;
#16842=CARTESIAN_POINT ( 'NONE',  ( -40.00000000000000711, 110.0000000000000000, -11.50000000000000000 ) ) ;
#16849=CARTESIAN_POINT ( 'NONE',  ( -24.00000000000000000, 53.00000000000000711, 30.00000000000000000 ) ) ;
#16851=ORIENTED_EDGE ( 'NONE', *, *, #2055, .F. ) ;
#16858=ORIENTED_EDGE ( 'NONE', *, *, #1135, .T. ) ;
#16871=DIRECTION ( 'NONE',  ( -1.156482317317871478E-16, 1.000000000000000000, 0.000000000000000000 ) ) ;
#16876=CARTESIAN_POINT ( 'NONE',  ( -40.00000000000000711, 113.0000000000000000, -18.00000000000000355 ) ) ;
#16878=CARTESIAN_POINT ( 'NONE',  ( -41.00000000000000711, 110.0000000000000000, -30.99999999999999645 ) ) ;
#16886=ORIENTED_EDGE ( 'NONE', *, *, #7318, .F. ) ;
#16894=CARTESIAN_POINT ( 'NONE',  ( -24.00000000000000711, 53.00000000000000711, -11.50000000000000000 ) ) ;
#16895=ORIENTED_EDGE ( 'NONE', *, *, #5203, .F. ) ;
#16896=DIRECTION ( 'NONE',  ( 1.000000000000000000, -0.000000000000000000, -0.000000000000000000 ) ) ;
#16903=VECTOR ( 'NONE', #7449, 1000.000000000000000 ) ;
#16904=CARTESIAN_POINT ( 'NONE',  ( -24.00000000000000000, 53.00000000000000711, -19.00000000000000355 ) ) ;
#16905=CARTESIAN_POINT ( 'NONE',  ( -41.00000000000000711, 113.0000000000000000, -50.00000000000000000 ) ) ;
#16906=LINE ( 'NONE', #6325, #9267 ) ;
#16907=VECTOR ( 'NONE', #2280, 1000.000000000000000 ) ;
#16913=VECTOR ( 'NONE', #16677, 1000.000000000000000 ) ;
#16915=EDGE_CURVE ( 'NONE', #1049, #3171, #622, .T. ) ;
#16935=ORIENTED_EDGE ( 'NONE', *, *, #9738, .T. ) ;
#16937=EDGE_CURVE ( 'NONE', #8366, #3614, #11007, .T. ) ;
#16948=VERTEX_POINT ( 'NONE', #8086 ) ;
#16955=VECTOR ( 'NONE', #14192, 1000.000000000000000 ) ;
#16957=EDGE_CURVE ( 'NONE', #6518, #11598, #2102, .T. ) ;
#16958=EDGE_CURVE ( 'NONE', #4628, #4224, #15330, .T. ) ;
#16959=DIRECTION ( 'NONE',  ( 1.156482317317871478E-16, -1.000000000000000000, 0.000000000000000000 ) ) ;
#16966=VECTOR ( 'NONE', #2857, 1000.000000000000000 ) ;
#16967=EDGE_LOOP ( 'NONE', ( #18820, #12518, #10441, #16121 ) ) ;
#16972=CARTESIAN_POINT ( 'NONE',  ( -41.00000000000000711, 110.0000000000000000, -24.49999999999999645 ) ) ;
#16973=ORIENTED_EDGE ( 'NONE', *, *, #10118, .T. ) ;
#16981=EDGE_CURVE ( 'NONE', #9587, #1661, #13756, .T. ) ;
#16982=FACE_OUTER_BOUND ( 'NONE', #14300, .T. ) ;
#16984=LINE ( 'NONE', #12453, #16766 ) ;
#16986=VECTOR ( 'NONE', #11862, 1000.000000000000000 ) ;
#16987=DIRECTION ( 'NONE',  ( 0.000000000000000000, -1.000000000000000000, 0.000000000000000000 ) ) ;
#16991=CARTESIAN_POINT ( 'NONE',  ( 0.000000000000000000, 0.000000000000000000, 30.00000000000000000 ) ) ;
#16999=ORIENTED_EDGE ( 'NONE', *, *, #11308, .F. ) ;
#17000=CARTESIAN_POINT ( 'NONE',  ( -32.50000000000000000, 52.00000000000000711, -37.65000000000000568 ) ) ;
#17005=DIRECTION ( 'NONE',  ( 1.000000000000000000, -0.000000000000000000, -0.000000000000000000 ) ) ;
#17006=VECTOR ( 'NONE', #2038, 1000.000000000000000 ) ;
#17007=CARTESIAN_POINT ( 'NONE',  ( -41.00000000000000711, 53.00000000000000711, -25.50000000000000000 ) ) ;
#17008=CARTESIAN_POINT ( 'NONE',  ( -24.00000000000000000, 53.00000000000000711, -11.49999999999999645 ) ) ;
#17012=ORIENTED_EDGE ( 'NONE', *, *, #3097, .F. ) ;
#17017=ADVANCED_FACE ( 'NONE', ( #16006, #2659, #8270, #15722, #13040, #3851, #8640, #14429, #10098, #9814, #11570, #6883, #8454 ), #3943, .F. ) ;
#17018=CARTESIAN_POINT ( 'NONE',  ( -24.00000000000000711, 53.00000000000000711, -19.00000000000000000 ) ) ;
#17021=PLANE ( 'NONE',  #7346 ) ;
#17026=CARTESIAN_POINT ( 'NONE',  ( -41.00000000000000711, 110.0000000000000000, -44.00000000000000000 ) ) ;
#17028=CARTESIAN_POINT ( 'NONE',  ( -41.00000000000000711, 53.00000000000000711, 6.999999999999999112 ) ) ;
#17031=VERTEX_POINT ( 'NONE', #6797 ) ;
#17040=LINE ( 'NONE', #9570, #4716 ) ;
#17050=VERTEX_POINT ( 'NONE', #4147 ) ;
#17055=ORIENTED_EDGE ( 'NONE', *, *, #14501, .T. ) ;
#17060=VECTOR ( 'NONE', #9829, 1000.000000000000000 ) ;
#17068=ORIENTED_EDGE ( 'NONE', *, *, #8741, .F. ) ;
#17073=CARTESIAN_POINT ( 'NONE',  ( -24.00000000000000000, 53.00000000000000711, 30.00000000000000000 ) ) ;
#17080=PLANE ( 'NONE',  #13307 ) ;
#17081=ORIENTED_EDGE ( 'NONE', *, *, #14772, .T. ) ;
#17086=EDGE_CURVE ( 'NONE', #12041, #184, #19038, .T. ) ;
#17089=VERTEX_POINT ( 'NONE', #12760 ) ;
#17091=CARTESIAN_POINT ( 'NONE',  ( -40.00000000000000711, 113.0000000000000000, -50.00000000000000000 ) ) ;
#17094=ADVANCED_FACE ( 'NONE', ( #18755 ), #8361, .T. ) ;
#17097=MANIFOLD_SOLID_BREP ( 'M5 Clearance Hole1', #19180 ) ;
#17108=DIRECTION ( 'NONE',  ( 1.000000000000000000, -0.000000000000000000, -0.000000000000000000 ) ) ;
#17119=LINE ( 'NONE', #2120, #15237 ) ;
#17124=AXIS2_PLACEMENT_3D ( 'NONE', #1475, #1276, #7344 ) ;
#17132=EDGE_LOOP ( 'NONE', ( #15701, #3116, #2748, #15439 ) ) ;
#17139=CARTESIAN_POINT ( 'NONE',  ( -41.00000000000000711, 53.00000000000000711, 21.00000000000000000 ) ) ;
#17140=LINE ( 'NONE', #3703, #9567 ) ;
#17146=ORIENTED_EDGE ( 'NONE', *, *, #4129, .F. ) ;
#17152=DIRECTION ( 'NONE',  ( 0.000000000000000000, -1.000000000000000000, 0.000000000000000000 ) ) ;
#17154=DIRECTION ( 'NONE',  ( 0.000000000000000000, -1.000000000000000000, -0.000000000000000000 ) ) ;
#17168=LINE ( 'NONE', #9703, #5342 ) ;
#17183=LINE ( 'NONE', #14420, #5940 ) ;
#17185=CARTESIAN_POINT ( 'NONE',  ( -41.00000000000000711, 53.00000000000000711, -44.00000000000000000 ) ) ;
#17187=VECTOR ( 'NONE', #14642, 1000.000000000000000 ) ;
#17189=EDGE_CURVE ( 'NONE', #13388, #2239, #13541, .T. ) ;
#17190=EDGE_CURVE ( 'NONE', #15646, #1350, #17964, .T. ) ;
#17191=CARTESIAN_POINT ( 'NONE',  ( -41.00000000000000711, 113.0000000000000000, 30.00000000000000000 ) ) ;
#17194=LINE ( 'NONE', #3946, #12403 ) ;
#17198=ADVANCED_FACE ( 'NONE', ( #10196 ), #11866, .T. ) ;
#17206=VECTOR ( 'NONE', #6785, 1000.000000000000000 ) ;
#17212=CARTESIAN_POINT ( 'NONE',  ( -41.00000000000000711, 53.00000000000000711, -24.49999999999999645 ) ) ;
#17213=VECTOR ( 'NONE', #1017, 1000.000000000000000 ) ;
#17214=VECTOR ( 'NONE', #15279, 1000.000000000000000 ) ;
#17233=DIRECTION ( 'NONE',  ( -1.000000000000000000, 0.000000000000000000, -0.000000000000000000 ) ) ;
#17238=VERTEX_POINT ( 'NONE', #13240 ) ;
#17241=ORIENTED_EDGE ( 'NONE', *, *, #4140, .T. ) ;
#17245=VECTOR ( 'NONE', #13427, 1000.000000000000000 ) ;
#17251=CARTESIAN_POINT ( 'NONE',  ( -24.00000000000000000, 113.0000000000000000, 30.00000000000000000 ) ) ;
#17252=VERTEX_POINT ( 'NONE', #11768 ) ;
#17275=PLANE ( 'NONE',  #3793 ) ;
#17278=LINE ( 'NONE', #9720, #4376 ) ;
#17281=DIRECTION ( 'NONE',  ( -1.156482317317871478E-16, 1.000000000000000000, 0.000000000000000000 ) ) ;
#17284=ADVANCED_FACE ( 'NONE', ( #9518 ), #17080, .T. ) ;
#17298=CARTESIAN_POINT ( 'NONE',  ( -25.00000000000000711, 53.00000000000000711, -38.50000000000000711 ) ) ;
#17300=EDGE_CURVE ( 'NONE', #17811, #853, #221, .T. ) ;
#17307=DIRECTION ( 'NONE',  ( 1.000000000000000000, -0.000000000000000000, -0.000000000000000000 ) ) ;
#17310=ORIENTED_EDGE ( 'NONE', *, *, #8459, .F. ) ;
#17314=CARTESIAN_POINT ( 'NONE',  ( -32.50000000000000000, 53.00000000000000711, 15.00000000000000000 ) ) ;
#17323=FACE_OUTER_BOUND ( 'NONE', #285, .T. ) ;
#17326=ORIENTED_EDGE ( 'NONE', *, *, #1582, .T. ) ;
#17330=ORIENTED_EDGE ( 'NONE', *, *, #5935, .F. ) ;
#17337=PLANE ( 'NONE',  #11241 ) ;
#17341=LINE ( 'NONE', #3910, #9392 ) ;
#17344=ADVANCED_FACE ( 'NONE', ( #15311 ), #12165, .F. ) ;
#17346=LINE ( 'NONE', #8421, #313 ) ;
#17349=CARTESIAN_POINT ( 'NONE',  ( -24.00000000000000000, 110.0000000000000000, 30.00000000000000000 ) ) ;
#17354=LINE ( 'NONE', #2547, #6480 ) ;
#17359=DIRECTION ( 'NONE',  ( 0.000000000000000000, -1.000000000000000000, -0.000000000000000000 ) ) ;
#17364=ORIENTED_EDGE ( 'NONE', *, *, #13525, .F. ) ;
#17365=CARTESIAN_POINT ( 'NONE',  ( -41.00000000000000711, 53.00000000000000711, -38.50000000000000711 ) ) ;
#17366=LINE ( 'NONE', #2283, #11108 ) ;
#17373=LINE ( 'NONE', #11673, #10500 ) ;
#17374=ORIENTED_EDGE ( 'NONE', *, *, #16937, .F. ) ;
#17382=CARTESIAN_POINT ( 'NONE',  ( -24.00000000000000000, 53.00000000000000711, 0.5000000000000004441 ) ) ;
#17389=CARTESIAN_POINT ( 'NONE',  ( -40.00000000000000000, 53.00000000000000711, 30.00000000000000000 ) ) ;
#17391=CARTESIAN_POINT ( 'NONE',  ( -41.00000000000000711, 53.00000000000000711, -44.00000000000000000 ) ) ;
#17394=VECTOR ( 'NONE', #4118, 1000.000000000000000 ) ;
#17412=CARTESIAN_POINT ( 'NONE',  ( -41.00000000000000711, 53.00000000000000711, 27.50000000000000000 ) ) ;
#17415=VECTOR ( 'NONE', #10080, 1000.000000000000000 ) ;
#17417=AXIS2_PLACEMENT_3D ( 'NONE', #12268, #1785, #16586 ) ;
#17435=LINE ( 'NONE', #3721, #626 ) ;
#17436=ORIENTED_EDGE ( 'NONE', *, *, #7719, .T. ) ;
#17445=ORIENTED_EDGE ( 'NONE', *, *, #10869, .F. ) ;
#17449=ORIENTED_EDGE ( 'NONE', *, *, #7605, .T. ) ;
#17453=ORIENTED_EDGE ( 'NONE', *, *, #8794, .T. ) ;
#17457=VERTEX_POINT ( 'NONE', #14497 ) ;
#17458=LINE ( 'NONE', #4030, #5323 ) ;
#17460=LINE ( 'NONE', #17562, #11917 ) ;
#17461=LINE ( 'NONE', #10291, #6003 ) ;
#17463=CARTESIAN_POINT ( 'NONE',  ( -41.00000000000000711, 53.00000000000000711, -19.00000000000000000 ) ) ;
#17471=VECTOR ( 'NONE', #3966, 1000.000000000000000 ) ;
#17472=DIRECTION ( 'NONE',  ( 0.000000000000000000, -1.000000000000000000, 0.000000000000000000 ) ) ;
#17473=VERTEX_POINT ( 'NONE', #2357 ) ;
#17488=ORIENTED_EDGE ( 'NONE', *, *, #8212, .T. ) ;
#17492=DIRECTION ( 'NONE',  ( 0.000000000000000000, 0.000000000000000000, 1.000000000000000000 ) ) ;
#17507=VECTOR ( 'NONE', #4521, 1000.000000000000000 ) ;
#17514=ORIENTED_EDGE ( 'NONE', *, *, #876, .F. ) ;
#17524=PLANE ( 'NONE',  #5661 ) ;
#17525=ORIENTED_EDGE ( 'NONE', *, *, #18416, .T. ) ;
#17530=ORIENTED_EDGE ( 'NONE', *, *, #9591, .T. ) ;
#17531=CARTESIAN_POINT ( 'NONE',  ( -24.00000000000000711, 110.0000000000000000, -44.00000000000000000 ) ) ;
#17538=PLANE ( 'NONE',  #14894 ) ;
#17542=ORIENTED_EDGE ( 'NONE', *, *, #6997, .F. ) ;
#17545=DIRECTION ( 'NONE',  ( 0.000000000000000000, -1.000000000000000000, 0.000000000000000000 ) ) ;
#17547=ORIENTED_EDGE ( 'NONE', *, *, #1479, .F. ) ;
#17552=EDGE_LOOP ( 'NONE', ( #5101, #16851, #7250, #9087 ) ) ;
#17555=ORIENTED_EDGE ( 'NONE', *, *, #13869, .F. ) ;
#17559=ORIENTED_EDGE ( 'NONE', *, *, #6743, .F. ) ;
#17560=CARTESIAN_POINT ( 'NONE',  ( -41.00000000000000711, 53.00000000000000711, -6.000000000000001776 ) ) ;
#17561=LINE ( 'NONE', #8268, #12377 ) ;
#17562=CARTESIAN_POINT ( 'NONE',  ( -24.00000000000000000, 110.0000000000000000, 30.00000000000000000 ) ) ;
#17563=VECTOR ( 'NONE', #2185, 1000.000000000000000 ) ;
#17575=VECTOR ( 'NONE', #3985, 1000.000000000000000 ) ;
#17582=ORIENTED_EDGE ( 'NONE', *, *, #16981, .T. ) ;
#17583=CARTESIAN_POINT ( 'NONE',  ( -24.00000000000000711, 53.00000000000000711, -5.000000000000000888 ) ) ;
#17586=CARTESIAN_POINT ( 'NONE',  ( -32.50000000000000000, 53.00000000000000711, -35.00000000000000000 ) ) ;
#17590=LINE ( 'NONE', #14450, #17187 ) ;
#17593=LINE ( 'NONE', #13262, #2381 ) ;
#17614=ORIENTED_EDGE ( 'NONE', *, *, #14769, .T. ) ;
#17620=PLANE ( 'NONE',  #67 ) ;
#17629=ORIENTED_EDGE ( 'NONE', *, *, #1106, .T. ) ;
#17634=CARTESIAN_POINT ( 'NONE',  ( -40.00000000000000711, 53.00000000000000711, -11.50000000000000000 ) ) ;
#17635=CARTESIAN_POINT ( 'NONE',  ( -41.00000000000000711, 110.0000000000000000, -24.49999999999999289 ) ) ;
#17638=VERTEX_POINT ( 'NONE', #14895 ) ;
#17642=VERTEX_POINT ( 'NONE', #8906 ) ;
#17652=VERTEX_POINT ( 'NONE', #16367 ) ;
#17656=CARTESIAN_POINT ( 'NONE',  ( -40.00000000000000000, 53.00000000000000711, -45.00000000000000000 ) ) ;
#17675=DIRECTION ( 'NONE',  ( -1.000000000000000000, 0.000000000000000000, -0.000000000000000000 ) ) ;
#17678=DIRECTION ( 'NONE',  ( 0.000000000000000000, 0.000000000000000000, -1.000000000000000000 ) ) ;
#17683=EDGE_CURVE ( 'NONE', #15895, #3842, #1369, .T. ) ;
#17686=CARTESIAN_POINT ( 'NONE',  ( -40.00000000000000000, 53.00000000000000711, 30.00000000000000000 ) ) ;
#17689=ORIENTED_EDGE ( 'NONE', *, *, #18170, .T. ) ;
#17698=CARTESIAN_POINT ( 'NONE',  ( -41.00000000000000711, 110.0000000000000000, -37.50000000000000711 ) ) ;
#17701=CARTESIAN_POINT ( 'NONE',  ( -40.00000000000000000, 53.00000000000000711, -25.50000000000000000 ) ) ;
#17702=CARTESIAN_POINT ( 'NONE',  ( -25.00000000000000711, 53.00000000000000711, -32.00000000000000000 ) ) ;
#17705=DIRECTION ( 'NONE',  ( 0.000000000000000000, 0.000000000000000000, 1.000000000000000000 ) ) ;
#17706=CARTESIAN_POINT ( 'NONE',  ( -41.00000000000000711, 110.0000000000000000, -6.000000000000001776 ) ) ;
#17722=ORIENTED_EDGE ( 'NONE', *, *, #7838, .F. ) ;
#17725=ORIENTED_EDGE ( 'NONE', *, *, #9053, .T. ) ;
#17727=CARTESIAN_POINT ( 'NONE',  ( -25.00000000000000000, 110.0000000000000000, -18.00000000000000355 ) ) ;
#17729=DIRECTION ( 'NONE',  ( -0.000000000000000000, -0.000000000000000000, -1.000000000000000000 ) ) ;
#17730=VECTOR ( 'NONE', #17545, 1000.000000000000000 ) ;
#17736=EDGE_LOOP ( 'NONE', ( #6876, #9394, #15299, #7329 ) ) ;
#17741=EDGE_CURVE ( 'NONE', #11533, #8015, #14989, .T. ) ;
#17747=VECTOR ( 'NONE', #2837, 1000.000000000000000 ) ;
#17749=LINE ( 'NONE', #10277, #16903 ) ;
#17751=ORIENTED_EDGE ( 'NONE', *, *, #15468, .T. ) ;
#17754=LINE ( 'NONE', #15006, #14744 ) ;
#17758=DIRECTION ( 'NONE',  ( 0.000000000000000000, -1.000000000000000000, -0.000000000000000000 ) ) ;
#17760=LINE ( 'NONE', #1685, #18827 ) ;
#17766=DIRECTION ( 'NONE',  ( -0.000000000000000000, -0.000000000000000000, -1.000000000000000000 ) ) ;
#17772=LINE ( 'NONE', #7283, #645 ) ;
#17778=LINE ( 'NONE', #4255, #634 ) ;
#17789=FACE_OUTER_BOUND ( 'NONE', #18114, .T. ) ;
#17791=VECTOR ( 'NONE', #16527, 1000.000000000000000 ) ;
#17800=EDGE_CURVE ( 'NONE', #12743, #9436, #12138, .T. ) ;
#17804=LINE ( 'NONE', #1534, #9655 ) ;
#17805=AXIS2_PLACEMENT_3D ( 'NONE', #9831, #11204, #735 ) ;
#17806=DIRECTION ( 'NONE',  ( -1.000000000000000000, 0.000000000000000000, -0.000000000000000000 ) ) ;
#17809=DIRECTION ( 'NONE',  ( 0.000000000000000000, 0.000000000000000000, -1.000000000000000000 ) ) ;
#17811=VERTEX_POINT ( 'NONE', #4810 ) ;
#17823=VERTEX_POINT ( 'NONE', #15190 ) ;
#17825=VERTEX_POINT ( 'NONE', #18038 ) ;
#17827=VERTEX_POINT ( 'NONE', #10566 ) ;
#17828=ORIENTED_EDGE ( 'NONE', *, *, #4305, .T. ) ;
#17830=DIRECTION ( 'NONE',  ( 0.000000000000000000, 0.000000000000000000, -1.000000000000000000 ) ) ;
#17838=VERTEX_POINT ( 'NONE', #4998 ) ;
#17839=ORIENTED_EDGE ( 'NONE', *, *, #3264, .T. ) ;
#17840=ORIENTED_EDGE ( 'NONE', *, *, #14178, .F. ) ;
#17845=ORIENTED_EDGE ( 'NONE', *, *, #8762, .F. ) ;
#17850=CARTESIAN_POINT ( 'NONE',  ( -25.00000000000000711, 53.00000000000000711, 26.50000000000000000 ) ) ;
#17854=VECTOR ( 'NONE', #18727, 1000.000000000000000 ) ;
#17857=LINE ( 'NONE', #16383, #11255 ) ;
#17859=LINE ( 'NONE', #15010, #15358 ) ;
#17864=VECTOR ( 'NONE', #8984, 1000.000000000000000 ) ;
#17873=VECTOR ( 'NONE', #5596, 1000.000000000000000 ) ;
#17876=DIRECTION ( 'NONE',  ( -0.000000000000000000, 1.000000000000000000, -0.000000000000000000 ) ) ;
#17878=VECTOR ( 'NONE', #14619, 1000.000000000000000 ) ;
#17879=CARTESIAN_POINT ( 'NONE',  ( -40.00000000000000000, 53.00000000000000711, -38.50000000000000711 ) ) ;
#17881=DIRECTION ( 'NONE',  ( 0.000000000000000000, 0.000000000000000000, -1.000000000000000000 ) ) ;
#17893=CARTESIAN_POINT ( 'NONE',  ( -41.00000000000000711, 53.00000000000000711, -5.000000000000000888 ) ) ;
#17894=VECTOR ( 'NONE', #13334, 1000.000000000000000 ) ;
#17895=ORIENTED_EDGE ( 'NONE', *, *, #4289, .F. ) ;
#17907=CARTESIAN_POINT ( 'NONE',  ( -41.00000000000000711, 110.0000000000000000, -32.00000000000000000 ) ) ;
#17912=DIRECTION ( 'NONE',  ( 0.000000000000000000, 0.000000000000000000, -1.000000000000000000 ) ) ;
#17917=EDGE_LOOP ( 'NONE', ( #4158, #692, #7086, #5138 ) ) ;
#17929=ORIENTED_EDGE ( 'NONE', *, *, #16480, .T. ) ;
#17935=PLANE ( 'NONE',  #1884 ) ;
#17944=CARTESIAN_POINT ( 'NONE',  ( -40.00000000000000000, 53.00000000000000711, 30.00000000000000000 ) ) ;
#17945=ORIENTED_EDGE ( 'NONE', *, *, #12293, .T. ) ;
#17955=CARTESIAN_POINT ( 'NONE',  ( -41.00000000000000711, 110.0000000000000000, -18.00000000000000000 ) ) ;
#17957=DIRECTION ( 'NONE',  ( 0.000000000000000000, 0.000000000000000000, -1.000000000000000000 ) ) ;
#17964=LINE ( 'NONE', #16392, #3315 ) ;
#17966=DIRECTION ( 'NONE',  ( 1.000000000000000000, -0.000000000000000000, -0.000000000000000000 ) ) ;
#17971=DIRECTION ( 'NONE',  ( 0.000000000000000000, -1.000000000000000000, 0.000000000000000000 ) ) ;
#17984=CARTESIAN_POINT ( 'NONE',  ( -25.00000000000000711, 53.00000000000000711, 6.999999999999999112 ) ) ;
#17985=ORIENTED_EDGE ( 'NONE', *, *, #3682, .T. ) ;
#17990=CARTESIAN_POINT ( 'NONE',  ( -24.00000000000000000, 53.00000000000000711, 26.50000000000000000 ) ) ;
#18019=CARTESIAN_POINT ( 'NONE',  ( -41.00000000000000711, 53.00000000000000711, -25.50000000000000000 ) ) ;
#18022=VECTOR ( 'NONE', #464, 1000.000000000000000 ) ;
#18025=VERTEX_POINT ( 'NONE', #18618 ) ;
#18033=ADVANCED_FACE ( 'NONE', ( #3989 ), #15947, .T. ) ;
#18035=LINE ( 'NONE', #7640, #4725 ) ;
#18038=CARTESIAN_POINT ( 'NONE',  ( -24.00000000000000711, 53.00000000000000711, -37.50000000000000711 ) ) ;
#18039=ORIENTED_EDGE ( 'NONE', *, *, #9548, .T. ) ;
#18040=ORIENTED_EDGE ( 'NONE', *, *, #13869, .T. ) ;
#18055=ORIENTED_EDGE ( 'NONE', *, *, #4744, .F. ) ;
#18058=EDGE_CURVE ( 'NONE', #3796, #1874, #17140, .T. ) ;
#18059=DIRECTION ( 'NONE',  ( 0.000000000000000000, 1.000000000000000000, 0.000000000000000000 ) ) ;
#18061=DIRECTION ( 'NONE',  ( 0.000000000000000000, -1.000000000000000000, 0.000000000000000000 ) ) ;
#18069=ORIENTED_EDGE ( 'NONE', *, *, #280, .F. ) ;
#18076=ORIENTED_EDGE ( 'NONE', *, *, #12291, .F. ) ;
#18077=LINE ( 'NONE', #10605, #9057 ) ;
#18079=EDGE_CURVE ( 'NONE', #19125, #6660, #14194, .T. ) ;
#18081=PLANE ( 'NONE',  #1077 ) ;
#18082=CARTESIAN_POINT ( 'NONE',  ( -40.00000000000000711, 53.00000000000000711, 27.50000000000000000 ) ) ;
#18100=EDGE_CURVE ( 'NONE', #9810, #13646, #12988, .T. ) ;
#18111=EDGE_CURVE ( 'NONE', #11, #9239, #11813, .T. ) ;
#18114=EDGE_LOOP ( 'NONE', ( #10653, #16973, #1510, #16233 ) ) ;
#18124=CARTESIAN_POINT ( 'NONE',  ( -40.00000000000000000, 53.00000000000000711, 30.00000000000000000 ) ) ;
#18130=DIRECTION ( 'NONE',  ( 1.000000000000000000, -0.000000000000000000, -0.000000000000000000 ) ) ;
#18132=DIRECTION ( 'NONE',  ( 0.000000000000000000, 1.000000000000000000, 0.000000000000000000 ) ) ;
#18134=VERTEX_POINT ( 'NONE', #1343 ) ;
#18137=VECTOR ( 'NONE', #9746, 1000.000000000000000 ) ;
#18139=EDGE_LOOP ( 'NONE', ( #509, #18179, #12273, #5559 ) ) ;
#18140=ORIENTED_EDGE ( 'NONE', *, *, #18079, .F. ) ;
#18147=EDGE_LOOP ( 'NONE', ( #15291, #1890, #13596, #11551 ) ) ;
#18148=EDGE_CURVE ( 'NONE', #1057, #4945, #19281, .T. ) ;
#18150=DIRECTION ( 'NONE',  ( -1.156482317317871478E-16, 1.000000000000000000, 0.000000000000000000 ) ) ;
#18154=DIRECTION ( 'NONE',  ( -1.156482317317871478E-16, 1.000000000000000000, 0.000000000000000000 ) ) ;
#18156=VECTOR ( 'NONE', #11112, 1000.000000000000000 ) ;
#18170=EDGE_CURVE ( 'NONE', #9366, #17827, #4087, .T. ) ;
#18172=VECTOR ( 'NONE', #10974, 1000.000000000000000 ) ;
#18179=ORIENTED_EDGE ( 'NONE', *, *, #14694, .T. ) ;
#18185=CIRCLE ( 'NONE', #1908, 2.649999999999999467 ) ;
#18198=LINE ( 'NONE', #13569, #10393 ) ;
#18201=LINE ( 'NONE', #60, #14535 ) ;
#18211=PLANE ( 'NONE',  #13632 ) ;
#18212=VECTOR ( 'NONE', #10976, 1000.000000000000000 ) ;
#18228=CARTESIAN_POINT ( 'NONE',  ( -41.00000000000000711, 53.00000000000000711, 26.50000000000000000 ) ) ;
#18234=CARTESIAN_POINT ( 'NONE',  ( -25.00000000000000000, 53.00000000000000711, -24.49999999999999289 ) ) ;
#18240=VECTOR ( 'NONE', #6524, 1000.000000000000000 ) ;
#18241=( NAMED_UNIT ( * ) SI_UNIT ( $, .STERADIAN. ) SOLID_ANGLE_UNIT ( ) );
#18243=ORIENTED_EDGE ( 'NONE', *, *, #1619, .F. ) ;
#18245=ADVANCED_FACE ( 'NONE', ( #1439 ), #2906, .F. ) ;
#18255=ORIENTED_EDGE ( 'NONE', *, *, #16837, .T. ) ;
#18258=CARTESIAN_POINT ( 'NONE',  ( -40.00000000000000711, 53.00000000000000711, 14.50000000000000000 ) ) ;
#18264=LINE ( 'NONE', #10783, #15988 ) ;
#18272=CARTESIAN_POINT ( 'NONE',  ( -41.00000000000000711, 53.00000000000000711, 1.500000000000001332 ) ) ;
#18273=VERTEX_POINT ( 'NONE', #18675 ) ;
#18278=VERTEX_POINT ( 'NONE', #3098 ) ;
#18288=LINE ( 'NONE', #16614, #6624 ) ;
#18296=DIRECTION ( 'NONE',  ( 0.000000000000000000, 0.000000000000000000, -1.000000000000000000 ) ) ;
#18302=EDGE_CURVE ( 'NONE', #11839, #17089, #6151, .T. ) ;
#18305=CARTESIAN_POINT ( 'NONE',  ( -41.00000000000000711, 110.0000000000000000, 27.50000000000000000 ) ) ;
#18310=ORIENTED_EDGE ( 'NONE', *, *, #16915, .T. ) ;
#18317=LINE ( 'NONE', #11038, #15534 ) ;
#18328=DIRECTION ( 'NONE',  ( -0.000000000000000000, -0.000000000000000000, -1.000000000000000000 ) ) ;
#18331=CARTESIAN_POINT ( 'NONE',  ( -41.00000000000000711, 53.00000000000000711, -19.00000000000000000 ) ) ;
#18334=ORIENTED_EDGE ( 'NONE', *, *, #18170, .F. ) ;
#18347=CARTESIAN_POINT ( 'NONE',  ( -40.00000000000000711, 113.0000000000000000, 21.00000000000000000 ) ) ;
#18355=VECTOR ( 'NONE', #10890, 1000.000000000000000 ) ;
#18358=VECTOR ( 'NONE', #13880, 1000.000000000000000 ) ;
#18359=FACE_OUTER_BOUND ( 'NONE', #3042, .T. ) ;
#18361=EDGE_CURVE ( 'NONE', #291, #6660, #13489, .T. ) ;
#18365=ORIENTED_EDGE ( 'NONE', *, *, #15060, .T. ) ;
#18368=LINE ( 'NONE', #18272, #18988 ) ;
#18377=LINE ( 'NONE', #332, #7175 ) ;
#18381=CARTESIAN_POINT ( 'NONE',  ( -41.00000000000000711, 110.0000000000000000, 13.50000000000000000 ) ) ;
#18387=FACE_OUTER_BOUND ( 'NONE', #5243, .T. ) ;
#18397=EDGE_CURVE ( 'NONE', #12335, #12613, #3667, .T. ) ;
#18416=EDGE_CURVE ( 'NONE', #12636, #8015, #14153, .T. ) ;
#18417=PLANE ( 'NONE',  #3316 ) ;
#18425=CARTESIAN_POINT ( 'NONE',  ( -40.00000000000000000, 53.00000000000000711, 30.00000000000000000 ) ) ;
#18436=EDGE_CURVE ( 'NONE', #10380, #2146, #17373, .T. ) ;
#18441=LINE ( 'NONE', #2153, #11881 ) ;
#18454=CARTESIAN_POINT ( 'NONE',  ( -32.50000000000000000, 53.00000000000000711, 12.35000000000000675 ) ) ;
#18490=VECTOR ( 'NONE', #14365, 1000.000000000000000 ) ;
#18503=DIRECTION ( 'NONE',  ( 1.000000000000000000, -0.000000000000000000, -0.000000000000000000 ) ) ;
#18508=ADVANCED_FACE ( 'NONE', ( #14525 ), #1096, .T. ) ;
#18520=ORIENTED_EDGE ( 'NONE', *, *, #15915, .F. ) ;
#18523=AXIS2_PLACEMENT_3D ( 'NONE', #14821, #2074, #15305 ) ;
#18525=CARTESIAN_POINT ( 'NONE',  ( -24.00000000000000000, 52.00000000000000711, -50.00000000000000000 ) ) ;
#18531=DIRECTION ( 'NONE',  ( 0.000000000000000000, -1.000000000000000000, -0.000000000000000000 ) ) ;
#18532=ORIENTED_EDGE ( 'NONE', *, *, #11425, .F. ) ;
#18533=ORIENTED_EDGE ( 'NONE', *, *, #9649, .F. ) ;
#18542=CARTESIAN_POINT ( 'NONE',  ( -41.00000000000000000, 52.00000000000000711, 30.00000000000000000 ) ) ;
#18555=DIRECTION ( 'NONE',  ( 0.000000000000000000, 0.000000000000000000, -1.000000000000000000 ) ) ;
#18569=CARTESIAN_POINT ( 'NONE',  ( -41.00000000000000711, 110.0000000000000000, 26.50000000000000000 ) ) ;
#18574=DIRECTION ( 'NONE',  ( 1.000000000000000000, -0.000000000000000000, -0.000000000000000000 ) ) ;
#18578=DIRECTION ( 'NONE',  ( 0.000000000000000000, 0.000000000000000000, -1.000000000000000000 ) ) ;
#18591=LINE ( 'NONE', #9269, #6538 ) ;
#18592=CARTESIAN_POINT ( 'NONE',  ( -32.50000000000000000, 52.00000000000000711, -35.00000000000000000 ) ) ;
#18593=CARTESIAN_POINT ( 'NONE',  ( -41.00000000000000711, 53.00000000000000711, -37.50000000000000711 ) ) ;
#18597=DIRECTION ( 'NONE',  ( 0.000000000000000000, 0.000000000000000000, -1.000000000000000000 ) ) ;
#18604=CARTESIAN_POINT ( 'NONE',  ( -25.00000000000000000, 110.0000000000000000, 1.500000000000001332 ) ) ;
#18605=EDGE_CURVE ( 'NONE', #7333, #13130, #8457, .T. ) ;
#18616=VECTOR ( 'NONE', #10908, 1000.000000000000000 ) ;
#18617=CARTESIAN_POINT ( 'NONE',  ( -41.00000000000000711, 53.00000000000000711, 0.5000000000000004441 ) ) ;
#18618=CARTESIAN_POINT ( 'NONE',  ( -24.00000000000000000, 110.0000000000000000, 0.5000000000000004441 ) ) ;
#18620=EDGE_CURVE ( 'NONE', #16642, #14902, #15024, .T. ) ;
#18623=( NAMED_UNIT ( * ) SI_UNIT ( $, .STERADIAN. ) SOLID_ANGLE_UNIT ( ) );
#18633=ORIENTED_EDGE ( 'NONE', *, *, #4704, .T. ) ;
#18653=EDGE_LOOP ( 'NONE', ( #9626, #12391 ) ) ;
#18664=VERTEX_POINT ( 'NONE', #9139 ) ;
#18665=VECTOR ( 'NONE', #18503, 1000.000000000000000 ) ;
#18666=CARTESIAN_POINT ( 'NONE',  ( -25.00000000000000000, 110.0000000000000000, -31.00000000000000000 ) ) ;
#18672=CARTESIAN_POINT ( 'NONE',  ( -25.00000000000000711, 110.0000000000000000, -19.00000000000000000 ) ) ;
#18675=CARTESIAN_POINT ( 'NONE',  ( -25.00000000000000711, 53.00000000000000711, -11.50000000000000000 ) ) ;
#18676=VECTOR ( 'NONE', #5634, 1000.000000000000000 ) ;
#18692=DIRECTION ( 'NONE',  ( 0.000000000000000000, 0.000000000000000000, 1.000000000000000000 ) ) ;
#18695=ORIENTED_EDGE ( 'NONE', *, *, #11623, .F. ) ;
#18697=VECTOR ( 'NONE', #16830, 1000.000000000000000 ) ;
#18700=CARTESIAN_POINT ( 'NONE',  ( -24.00000000000000000, 53.00000000000000711, -6.000000000000005329 ) ) ;
#18703=ORIENTED_EDGE ( 'NONE', *, *, #5467, .F. ) ;
#18707=LINE ( 'NONE', #670, #612 ) ;
#18725=DIRECTION ( 'NONE',  ( 0.000000000000000000, 0.000000000000000000, -1.000000000000000000 ) ) ;
#18727=DIRECTION ( 'NONE',  ( -0.000000000000000000, -0.000000000000000000, -1.000000000000000000 ) ) ;
#18732=DIRECTION ( 'NONE',  ( 0.000000000000000000, 0.000000000000000000, -1.000000000000000000 ) ) ;
#18736=DIRECTION ( 'NONE',  ( 0.000000000000000000, 0.000000000000000000, -1.000000000000000000 ) ) ;
#18747=CARTESIAN_POINT ( 'NONE',  ( -41.00000000000000711, 53.00000000000000711, -37.50000000000000711 ) ) ;
#18751=ORIENTED_EDGE ( 'NONE', *, *, #3395, .F. ) ;
#18754=CARTESIAN_POINT ( 'NONE',  ( -24.00000000000000711, 110.0000000000000000, 27.50000000000000000 ) ) ;
#18755=FACE_OUTER_BOUND ( 'NONE', #13625, .T. ) ;
#18760=ORIENTED_EDGE ( 'NONE', *, *, #4645, .F. ) ;
#18761=VECTOR ( 'NONE', #1532, 1000.000000000000000 ) ;
#18770=PLANE ( 'NONE',  #17805 ) ;
#18779=CARTESIAN_POINT ( 'NONE',  ( -24.00000000000000000, 53.00000000000000711, 13.49999999999999822 ) ) ;
#18781=ORIENTED_EDGE ( 'NONE', *, *, #12291, .T. ) ;
#18785=DIRECTION ( 'NONE',  ( 0.000000000000000000, -1.000000000000000000, 0.000000000000000000 ) ) ;
#18789=ORIENTED_EDGE ( 'NONE', *, *, #18302, .T. ) ;
#18790=LINE ( 'NONE', #6824, #18490 ) ;
#18807=VERTEX_POINT ( 'NONE', #12568 ) ;
#18820=ORIENTED_EDGE ( 'NONE', *, *, #7198, .T. ) ;
#18822=FACE_OUTER_BOUND ( 'NONE', #2871, .T. ) ;
#18823=DIRECTION ( 'NONE',  ( -0.000000000000000000, 1.000000000000000000, -0.000000000000000000 ) ) ;
#18825=VECTOR ( 'NONE', #16155, 1000.000000000000000 ) ;
#18827=VECTOR ( 'NONE', #6002, 1000.000000000000000 ) ;
#18834=EDGE_CURVE ( 'NONE', #13602, #2358, #3363, .T. ) ;
#18836=CARTESIAN_POINT ( 'NONE',  ( -41.00000000000000711, 110.0000000000000000, 8.000000000000000000 ) ) ;
#18840=PLANE ( 'NONE',  #5611 ) ;
#18853=EDGE_CURVE ( 'NONE', #9106, #17089, #3553, .T. ) ;
#18854=EDGE_CURVE ( 'NONE', #17823, #2170, #18368, .T. ) ;
#18861=ORIENTED_EDGE ( 'NONE', *, *, #13459, .T. ) ;
#18863=ORIENTED_EDGE ( 'NONE', *, *, #6865, .T. ) ;
#18876=ADVANCED_FACE ( 'NONE', ( #2172 ), #15423, .F. ) ;
#18892=DIRECTION ( 'NONE',  ( 0.000000000000000000, 1.000000000000000000, 0.000000000000000000 ) ) ;
#18896=CARTESIAN_POINT ( 'NONE',  ( -41.00000000000000711, 53.00000000000000711, 6.999999999999999112 ) ) ;
#18909=ORIENTED_EDGE ( 'NONE', *, *, #16580, .T. ) ;
#18913=VERTEX_POINT ( 'NONE', #10793 ) ;
#18931=CARTESIAN_POINT ( 'NONE',  ( -41.00000000000000711, 110.0000000000000000, -12.50000000000000000 ) ) ;
#18936=EDGE_CURVE ( 'NONE', #17652, #982, #16161, .T. ) ;
#18940=DIRECTION ( 'NONE',  ( 0.000000000000000000, 0.000000000000000000, -1.000000000000000000 ) ) ;
#18965=VECTOR ( 'NONE', #8551, 1000.000000000000000 ) ;
#18966=VECTOR ( 'NONE', #13680, 1000.000000000000000 ) ;
#18968=FACE_OUTER_BOUND ( 'NONE', #15982, .T. ) ;
#18974=EDGE_CURVE ( 'NONE', #8044, #1767, #3261, .T. ) ;
#18980=AXIS2_PLACEMENT_3D ( 'NONE', #5833, #7194, #13169 ) ;
#18988=VECTOR ( 'NONE', #13844, 1000.000000000000000 ) ;
#18991=EDGE_CURVE ( 'NONE', #10947, #10091, #16074, .T. ) ;
#18992=ORIENTED_EDGE ( 'NONE', *, *, #6763, .F. ) ;
#18996=FILL_AREA_STYLE ('',( #952 ) ) ;
#18998=VERTEX_POINT ( 'NONE', #18836 ) ;
#18999=VERTEX_POINT ( 'NONE', #6862 ) ;
#19004=FACE_OUTER_BOUND ( 'NONE', #11963, .T. ) ;
#19005=VERTEX_POINT ( 'NONE', #5493 ) ;
#19007=CARTESIAN_POINT ( 'NONE',  ( -41.00000000000000711, 53.00000000000000711, -44.00000000000000000 ) ) ;
#19026=FACE_OUTER_BOUND ( 'NONE', #17736, .T. ) ;
#19031=FACE_OUTER_BOUND ( 'NONE', #7761, .T. ) ;
#19032=ORIENTED_EDGE ( 'NONE', *, *, #11695, .F. ) ;
#19034=CARTESIAN_POINT ( 'NONE',  ( -40.00000000000000711, 113.0000000000000000, -25.49999999999999645 ) ) ;
#19035=DIRECTION ( 'NONE',  ( 0.000000000000000000, 0.000000000000000000, 1.000000000000000000 ) ) ;
#19038=LINE ( 'NONE', #8548, #7007 ) ;
#19039=EDGE_CURVE ( 'NONE', #2835, #17031, #17354, .T. ) ;
#19049=ORIENTED_EDGE ( 'NONE', *, *, #6024, .F. ) ;
#19061=CARTESIAN_POINT ( 'NONE',  ( -40.00000000000000711, 110.0000000000000000, 30.00000000000000000 ) ) ;
#19064=EDGE_CURVE ( 'NONE', #10051, #13646, #9710, .T. ) ;
#19068=DIRECTION ( 'NONE',  ( -1.000000000000000000, 0.000000000000000000, -0.000000000000000000 ) ) ;
#19077=LINE ( 'NONE', #2798, #19382 ) ;
#19078=PLANE ( 'NONE',  #6828 ) ;
#19079=CARTESIAN_POINT ( 'NONE',  ( -24.00000000000000711, 53.00000000000000711, 6.999999999999999112 ) ) ;
#19082=LINE ( 'NONE', #12799, #2529 ) ;
#19083=EDGE_CURVE ( 'NONE', #11529, #1874, #3925, .T. ) ;
#19085=CARTESIAN_POINT ( 'NONE',  ( -41.00000000000000711, 53.00000000000000711, -38.50000000000000711 ) ) ;
#19092=ORIENTED_EDGE ( 'NONE', *, *, #8903, .F. ) ;
#19110=ADVANCED_FACE ( 'NONE', ( #4126 ), #5589, .F. ) ;
#19125=VERTEX_POINT ( 'NONE', #12930 ) ;
#19128=VERTEX_POINT ( 'NONE', #3738 ) ;
#19131=EDGE_LOOP ( 'NONE', ( #7694, #17725, #9059, #10274 ) ) ;
#19133=CARTESIAN_POINT ( 'NONE',  ( -40.00000000000000711, 110.0000000000000000, -32.00000000000000000 ) ) ;
#19144=ORIENTED_EDGE ( 'NONE', *, *, #7485, .F. ) ;
#19147=VECTOR ( 'NONE', #3390, 1000.000000000000000 ) ;
#19153=ORIENTED_EDGE ( 'NONE', *, *, #11675, .F. ) ;
#19155=PLANE ( 'NONE',  #7817 ) ;
#19162=CARTESIAN_POINT ( 'NONE',  ( -25.00000000000000711, 53.00000000000000711, -25.50000000000000000 ) ) ;
#19178=EDGE_CURVE ( 'NONE', #2911, #1370, #15984, .T. ) ;
#19179=CARTESIAN_POINT ( 'NONE',  ( -41.00000000000000711, 53.00000000000000711, 20.00000000000000000 ) ) ;
#19180=CLOSED_SHELL ( 'NONE', ( #4870, #16113, #14355, #11286, #9971, #16803, #453, #17094, #17017, #1342, #17344, #15749, #10194, #13862, #8307, #18876, #11612, #10847, #12817, #6571, #7253, #3178, #16457, #3648, #1196, #13608, #15530, #3039, #19240, #7777, #14585, #7931, #13477, #617, #16220, #19110, #12276, #3777, #6721, #15572, #3735, #1006, #4236, #18508, #8939, #15378, #13304, #14866, #3254, #16422, #8061, #15041, #2106, #6738, #18245, #4786, #897, #3399, #6248, #15767, #10896, #14665, #3023, #14722, #11643, #16204, #7197, #10784, #5120, #12855, #16031, #5766, #12153, #8637, #18033, #8085, #1616, #5056, #6667, #17198, #17284, #8184, #9525, #4133, #16612, #2844 ) ) ;
#19182=LINE ( 'NONE', #14963, #3174 ) ;
#19204=LINE ( 'NONE', #15091, #17214 ) ;
#19208=LINE ( 'NONE', #3918, #4576 ) ;
#19212=ORIENTED_EDGE ( 'NONE', *, *, #18397, .T. ) ;
#19215=VERTEX_POINT ( 'NONE', #17944 ) ;
#19220=LINE ( 'NONE', #6086, #17507 ) ;
#19225=ORIENTED_EDGE ( 'NONE', *, *, #13088, .T. ) ;
#19227=ORIENTED_EDGE ( 'NONE', *, *, #13190, .T. ) ;
#19240=ADVANCED_FACE ( 'NONE', ( #13120 ), #13521, .T. ) ;
#19248=VERTEX_POINT ( 'NONE', #4217 ) ;
#19263=EDGE_CURVE ( 'NONE', #18664, #17089, #8911, .T. ) ;
#19264=ORIENTED_EDGE ( 'NONE', *, *, #12226, .F. ) ;
#19281=LINE ( 'NONE', #17706, #1117 ) ;
#19282=ORIENTED_EDGE ( 'NONE', *, *, #5521, .T. ) ;
#19283=VERTEX_POINT ( 'NONE', #2324 ) ;
#19287=LINE ( 'NONE', #14971, #17864 ) ;
#19288=ORIENTED_EDGE ( 'NONE', *, *, #9244, .T. ) ;
#19301=ORIENTED_EDGE ( 'NONE', *, *, #12009, .F. ) ;
#19311=ORIENTED_EDGE ( 'NONE', *, *, #5642, .F. ) ;
#19312=EDGE_LOOP ( 'NONE', ( #5308, #1939, #12341, #8142 ) ) ;
#19320=CARTESIAN_POINT ( 'NONE',  ( -41.00000000000000711, 110.0000000000000000, -24.49999999999999645 ) ) ;
#19321=CARTESIAN_POINT ( 'NONE',  ( -41.00000000000000711, 53.00000000000000711, -25.50000000000000000 ) ) ;
#19324=CARTESIAN_POINT ( 'NONE',  ( -41.00000000000000711, 53.00000000000000711, -19.00000000000000000 ) ) ;
#19328=DIRECTION ( 'NONE',  ( 1.000000000000000000, -0.000000000000000000, -0.000000000000000000 ) ) ;
#19330=CARTESIAN_POINT ( 'NONE',  ( -41.00000000000000711, 53.00000000000000711, -25.50000000000000000 ) ) ;
#19334=DIRECTION ( 'NONE',  ( 1.000000000000000000, 0.000000000000000000, 0.000000000000000000 ) ) ;
#19336=DIRECTION ( 'NONE',  ( -0.000000000000000000, -0.000000000000000000, -1.000000000000000000 ) ) ;
#19345=DIRECTION ( 'NONE',  ( 1.000000000000000000, -0.000000000000000000, -0.000000000000000000 ) ) ;
#19353=LINE ( 'NONE', #4848, #7214 ) ;
#19358=DIRECTION ( 'NONE',  ( 0.000000000000000000, 0.000000000000000000, 1.000000000000000000 ) ) ;
#19372=LINE ( 'NONE', #254, #5588 ) ;
#19375=FACE_OUTER_BOUND ( 'NONE', #5218, .T. ) ;
#19378=ORIENTED_EDGE ( 'NONE', *, *, #4171, .T. ) ;
#19382=VECTOR ( 'NONE', #11808, 1000.000000000000000 ) ;
#19393=DIRECTION ( 'NONE',  ( 1.000000000000000000, -0.000000000000000000, -0.000000000000000000 ) ) ;
#19394=VERTEX_POINT ( 'NONE', #2049 ) ;
ENDSEC;
END-ISO-10303-21;
